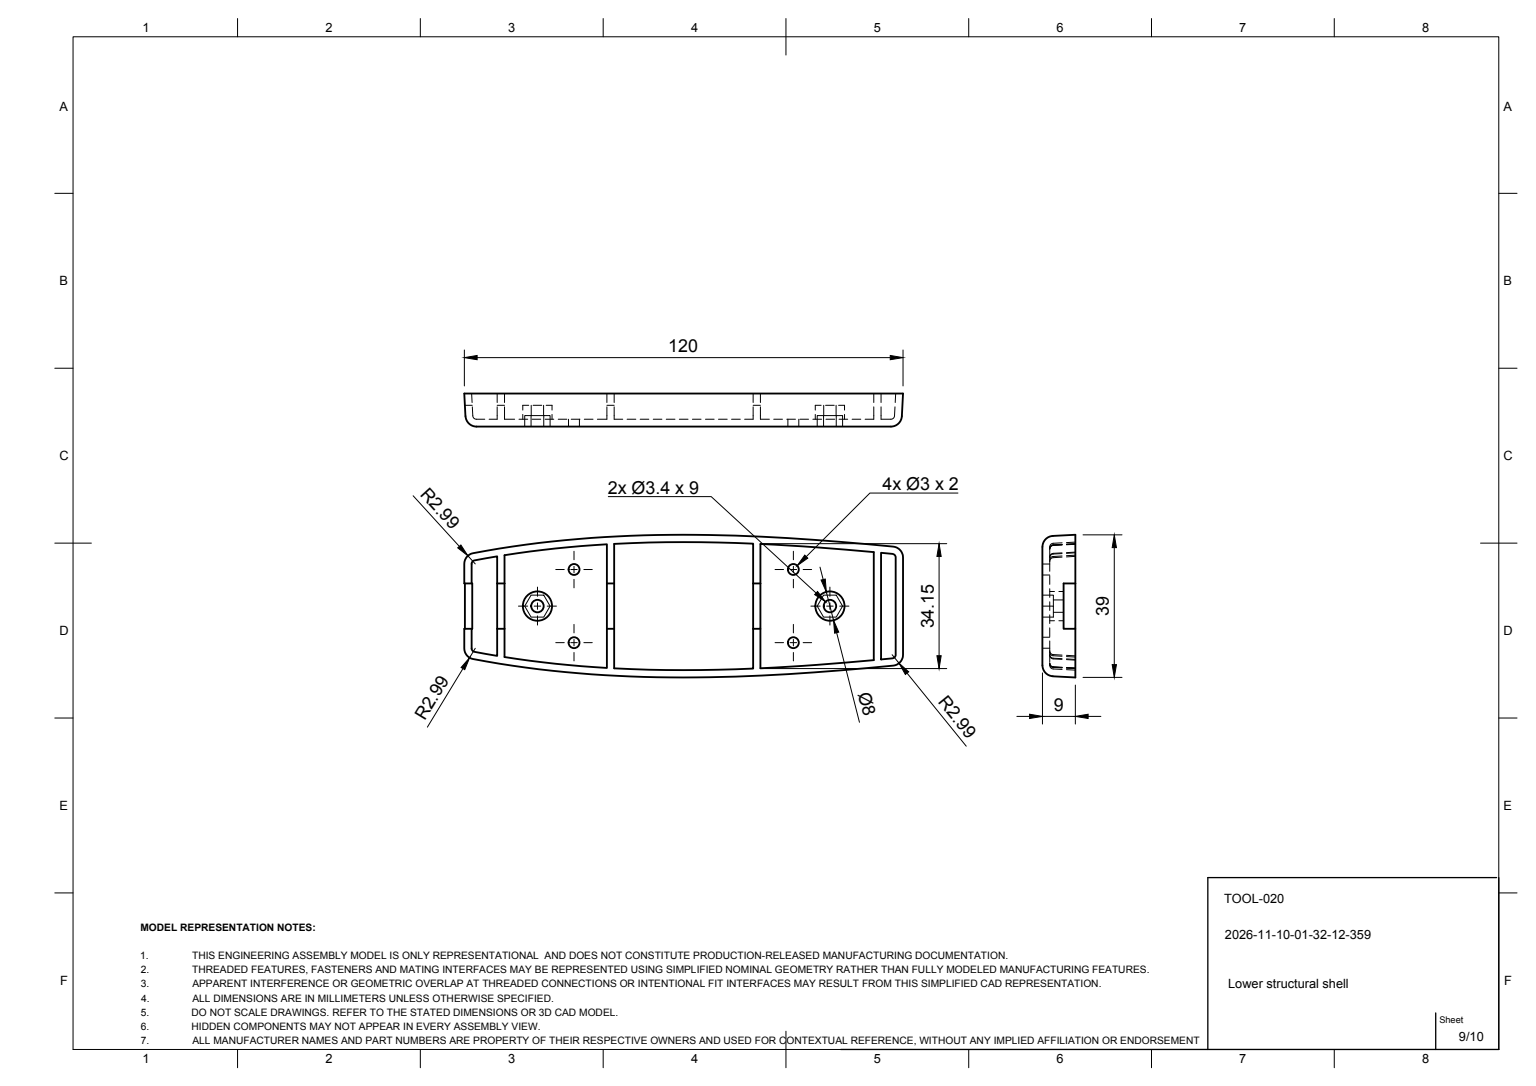
ISO-10303-21;
HEADER;
/* Generated by software containing ST-Developer
 * from STEP Tools, Inc. (www.steptools.com) 
 */

FILE_DESCRIPTION(
/* description */ (''),
/* implementation_level */ '2;1');

FILE_NAME(
/* name */ 'Lower structural shell.step',
/* time_stamp */ '2026-11-10T09:09:39-08:00',
/* author */ (''),
/* organization */ (''),
/* preprocessor_version */ 'ST-DEVELOPER v20.2',
/* originating_system */ 'Autodesk Translation Framework v15.17.0.0',
/* authorisation */ '');

FILE_SCHEMA (('AUTOMOTIVE_DESIGN { 1 0 10303 214 3 1 1 }'));
ENDSEC;

DATA;
#10=MECHANICAL_DESIGN_GEOMETRIC_PRESENTATION_REPRESENTATION('',(#559),#18353);
#83=SPHERICAL_SURFACE('',#6859,0.0999999999999999);
#84=SPHERICAL_SURFACE('',#6862,0.100000000000002);
#85=SPHERICAL_SURFACE('',#6866,0.0999999999999991);
#86=SPHERICAL_SURFACE('',#6870,0.1);
#87=SPHERICAL_SURFACE('',#6875,0.3);
#88=SPHERICAL_SURFACE('',#6879,0.300000000000002);
#89=SPHERICAL_SURFACE('',#6883,0.299999999999999);
#90=SPHERICAL_SURFACE('',#6888,0.3);
#123=B_SPLINE_SURFACE_WITH_KNOTS('',3,3,((#11565,#11566,#11567,#11568),
(#11569,#11570,#11571,#11572),(#11573,#11574,#11575,#11576),(#11577,#11578,
#11579,#11580)),.UNSPECIFIED.,.F.,.F.,.F.,(4,4),(4,4),(0.0627625298587661,
0.3242096015809),(0.0118073085896899,0.685451490706028),.UNSPECIFIED.);
#124=B_SPLINE_SURFACE_WITH_KNOTS('',3,3,((#11585,#11586,#11587,#11588),
(#11589,#11590,#11591,#11592),(#11593,#11594,#11595,#11596),(#11597,#11598,
#11599,#11600)),.UNSPECIFIED.,.F.,.F.,.F.,(4,4),(4,4),(0.0225360950145449,
0.0483865590996774),(0.0125659096559557,0.685650832343257),
 .UNSPECIFIED.);
#125=B_SPLINE_SURFACE_WITH_KNOTS('',3,3,((#11610,#11611,#11612,#11613),
(#11614,#11615,#11616,#11617),(#11618,#11619,#11620,#11621),(#11622,#11623,
#11624,#11625),(#11626,#11627,#11628,#11629)),.UNSPECIFIED.,.F.,.F.,.F.,
(4,1,4),(4,4),(0.,0.571428571428571,1.),(0.74118252158834,3.85438678954986),
 .UNSPECIFIED.);
#126=B_SPLINE_SURFACE_WITH_KNOTS('',3,3,((#11634,#11635,#11636,#11637),
(#11638,#11639,#11640,#11641),(#11642,#11643,#11644,#11645),(#11646,#11647,
#11648,#11649),(#11650,#11651,#11652,#11653)),.UNSPECIFIED.,.F.,.F.,.F.,
(4,1,4),(4,4),(0.,0.571428571428571,1.),(0.270878787657975,0.54981857912664),
 .UNSPECIFIED.);
#127=B_SPLINE_SURFACE_WITH_KNOTS('',3,3,((#11672,#11673,#11674,#11675),
(#11676,#11677,#11678,#11679),(#11680,#11681,#11682,#11683),(#11684,#11685,
#11686,#11687),(#11688,#11689,#11690,#11691)),.UNSPECIFIED.,.F.,.F.,.F.,
(4,1,4),(4,4),(0.,0.571428571428571,1.),(8.03948512627517,11.1526893942367),
 .UNSPECIFIED.);
#128=B_SPLINE_SURFACE_WITH_KNOTS('',3,3,((#11696,#11697,#11698,#11699),
(#11700,#11701,#11702,#11703),(#11704,#11705,#11706,#11707),(#11708,#11709,
#11710,#11711)),.UNSPECIFIED.,.F.,.F.,.F.,(4,4),(4,4),(0.675790398419059,
0.937237470141233),(0.0118073085603101,0.685451490706029),.UNSPECIFIED.);
#129=B_SPLINE_SURFACE_WITH_KNOTS('',3,3,((#11712,#11713,#11714,#11715),
(#11716,#11717,#11718,#11719),(#11720,#11721,#11722,#11723),(#11724,#11725,
#11726,#11727)),.UNSPECIFIED.,.F.,.F.,.F.,(4,4),(4,4),(0.951613440900322,
0.977463904985455),(0.0125659096559558,0.685650832343257),.UNSPECIFIED.);
#130=B_SPLINE_SURFACE_WITH_KNOTS('',3,3,((#11811,#11812,#11813,#11814),
(#11815,#11816,#11817,#11818),(#11819,#11820,#11821,#11822),(#11823,#11824,
#11825,#11826)),.UNSPECIFIED.,.F.,.F.,.F.,(4,4),(4,4),(0.340089900275858,
0.660082688299826),(0.0116294244283504,0.684384408933581),.UNSPECIFIED.);
#131=B_SPLINE_SURFACE_WITH_KNOTS('',3,3,((#11831,#11832,#11833,#11834),
(#11835,#11836,#11837,#11838),(#11839,#11840,#11841,#11842),(#11843,#11844,
#11845,#11846),(#11847,#11848,#11849,#11850)),.UNSPECIFIED.,.F.,.F.,.F.,
(4,1,4),(4,4),(0.,0.571428571428571,1.),(4.04989375377528,7.85140214144331),
 .UNSPECIFIED.);
#132=B_SPLINE_SURFACE_WITH_KNOTS('',3,3,((#11860,#11861,#11862,#11863),
(#11864,#11865,#11866,#11867),(#11868,#11869,#11870,#11871),(#11872,#11873,
#11874,#11875),(#11876,#11877,#11878,#11879)),.UNSPECIFIED.,.F.,.F.,.F.,
(4,1,4),(4,4),(0.,0.571428571428571,1.),(4.0424697743818,7.84397816204974),
 .UNSPECIFIED.);
#133=B_SPLINE_SURFACE_WITH_KNOTS('',3,3,((#11884,#11885,#11886,#11887),
(#11888,#11889,#11890,#11891),(#11892,#11893,#11894,#11895),(#11896,#11897,
#11898,#11899)),.UNSPECIFIED.,.F.,.F.,.F.,(4,4),(4,4),(0.339917311700174,
0.659910099724142),(0.0116294573698948,0.684384408933581),.UNSPECIFIED.);
#134=B_SPLINE_SURFACE_WITH_KNOTS('',3,3,((#11974,#11975,#11976,#11977),
(#11978,#11979,#11980,#11981),(#11982,#11983,#11984,#11985),(#11986,#11987,
#11988,#11989)),.UNSPECIFIED.,.F.,.F.,.F.,(4,4),(4,4),(0.675996615945502,
0.913173856075534),(0.0118505108223707,0.686152089762332),.UNSPECIFIED.);
#135=B_SPLINE_SURFACE_WITH_KNOTS('',3,3,((#11994,#11995,#11996,#11997),
(#11998,#11999,#12000,#12001),(#12002,#12003,#12004,#12005),(#12006,#12007,
#12008,#12009),(#12010,#12011,#12012,#12013)),.UNSPECIFIED.,.F.,.F.,.F.,
(4,1,4),(4,4),(0.,0.571428571428571,1.),(8.0457708503995,10.8690635835914),
 .UNSPECIFIED.);
#136=B_SPLINE_SURFACE_WITH_KNOTS('',3,3,((#12023,#12024,#12025,#12026),
(#12027,#12028,#12029,#12030),(#12031,#12032,#12033,#12034),(#12035,#12036,
#12037,#12038),(#12039,#12040,#12041,#12042)),.UNSPECIFIED.,.F.,.F.,.F.,
(4,1,4),(4,4),(0.,0.571428571428571,1.),(1.02480833223363,3.8481010654256),
 .UNSPECIFIED.);
#137=B_SPLINE_SURFACE_WITH_KNOTS('',3,3,((#12047,#12048,#12049,#12050),
(#12051,#12052,#12053,#12054),(#12055,#12056,#12057,#12058),(#12059,#12060,
#12061,#12062)),.UNSPECIFIED.,.F.,.F.,.F.,(4,4),(4,4),(0.0868261439244655,
0.324003384054498),(0.0118505108223707,0.686152089762332),.UNSPECIFIED.);
#138=B_SPLINE_SURFACE_WITH_KNOTS('',3,3,((#12137,#12138,#12139,#12140),
(#12141,#12142,#12143,#12144),(#12145,#12146,#12147,#12148),(#12149,#12150,
#12151,#12152)),.UNSPECIFIED.,.F.,.F.,.F.,(4,4),(4,4),(0.927751606342899,
0.979699913047832),(0.0130895688562318,0.686930956013783),.UNSPECIFIED.);
#139=B_SPLINE_SURFACE_WITH_KNOTS('',3,3,((#12162,#12163,#12164,#12165),
(#12166,#12167,#12168,#12169),(#12170,#12171,#12172,#12173),(#12174,#12175,
#12176,#12177),(#12178,#12179,#12180,#12181)),.UNSPECIFIED.,.F.,.F.,.F.,
(4,1,4),(4,4),(0.,0.571428571428571,1.),(11.0550486447215,11.6488871259622),
 .UNSPECIFIED.);
#140=B_SPLINE_SURFACE_WITH_KNOTS('',3,3,((#12195,#12196,#12197,#12198),
(#12199,#12200,#12201,#12202),(#12203,#12204,#12205,#12206),(#12207,#12208,
#12209,#12210)),.UNSPECIFIED.,.F.,.F.,.F.,(4,4),(4,4),(0.0203000869521683,
0.0722483936571013),(0.0130895688562318,0.686930956013783),
 .UNSPECIFIED.);
#141=B_SPLINE_SURFACE_WITH_KNOTS('',3,3,((#12220,#12221,#12222,#12223),
(#12224,#12225,#12226,#12227),(#12228,#12229,#12230,#12231),(#12232,#12233,
#12234,#12235),(#12236,#12237,#12238,#12239)),.UNSPECIFIED.,.F.,.F.,.F.,
(4,1,4),(4,4),(0.,0.571428571428571,1.),(0.244984789862841,0.838823271103535),
 .UNSPECIFIED.);
#142=B_SPLINE_SURFACE_WITH_KNOTS('',3,3,((#12253,#12254,#12255,#12256),
(#12257,#12258,#12259,#12260),(#12261,#12262,#12263,#12264),(#12265,#12266,
#12267,#12268),(#12269,#12270,#12271,#12272)),.UNSPECIFIED.,.F.,.F.,.F.,
(4,1,4),(4,4),(0.,0.5,1.),(0.0108921325678979,0.619909717328002),
 .UNSPECIFIED.);
#143=B_SPLINE_SURFACE_WITH_KNOTS('',3,3,((#12279,#12280,#12281,#12282),
(#12283,#12284,#12285,#12286),(#12287,#12288,#12289,#12290),(#12291,#12292,
#12293,#12294),(#12295,#12296,#12297,#12298)),.UNSPECIFIED.,.F.,.F.,.F.,
(4,1,4),(4,4),(0.,0.571428571428571,1.),(0.00967450486392679,0.618764321025346),
 .UNSPECIFIED.);
#144=B_SPLINE_SURFACE_WITH_KNOTS('',3,3,((#12303,#12304,#12305,#12306),
(#12307,#12308,#12309,#12310),(#12311,#12312,#12313,#12314),(#12315,#12316,
#12317,#12318),(#12319,#12320,#12321,#12322)),.UNSPECIFIED.,.F.,.F.,.F.,
(4,1,4),(4,4),(0.,0.571428571428571,1.),(0.0097274579809394,0.618764321025346),
 .UNSPECIFIED.);
#145=B_SPLINE_SURFACE_WITH_KNOTS('',3,3,((#12327,#12328,#12329,#12330),
(#12331,#12332,#12333,#12334),(#12335,#12336,#12337,#12338),(#12339,#12340,
#12341,#12342),(#12343,#12344,#12345,#12346)),.UNSPECIFIED.,.F.,.F.,.F.,
(4,1,4),(4,4),(0.,0.571428571428571,1.),(11.3440533366984,11.6229931281671),
 .UNSPECIFIED.);
#146=B_SPLINE_SURFACE_WITH_KNOTS('',3,3,((#12347,#12348,#12349,#12350),
(#12351,#12352,#12353,#12354),(#12355,#12356,#12357,#12358),(#12359,#12360,
#12361,#12362),(#12363,#12364,#12365,#12366)),.UNSPECIFIED.,.F.,.F.,.F.,
(4,1,4),(4,4),(0.,0.5,1.),(0.0108402259132964,0.619909717328002),
 .UNSPECIFIED.);
#147=B_SPLINE_SURFACE_WITH_KNOTS('',3,3,((#12392,#12393,#12394,#12395),
(#12396,#12397,#12398,#12399),(#12400,#12401,#12402,#12403),(#12404,#12405,
#12406,#12407),(#12408,#12409,#12410,#12411)),.UNSPECIFIED.,.F.,.F.,.F.,
(4,1,4),(4,4),(0.,0.571428571428571,1.),(-0.00387706229521417,0.619909717328002),
 .UNSPECIFIED.);
#148=B_SPLINE_SURFACE_WITH_KNOTS('',3,3,((#12430,#12431,#12432,#12433,#12434,
#12435),(#12436,#12437,#12438,#12439,#12440,#12441),(#12442,#12443,#12444,
#12445,#12446,#12447),(#12448,#12449,#12450,#12451,#12452,#12453),(#12454,
#12455,#12456,#12457,#12458,#12459)),.UNSPECIFIED.,.F.,.F.,.F.,(4,1,4),
(4,1,1,4),(0.,0.571428571428571,1.),(0.270878787657975,5.14716807550265,
8.39802760073243,11.6488871259622),.UNSPECIFIED.);
#149=B_SPLINE_SURFACE_WITH_KNOTS('',3,3,((#12472,#12473,#12474,#12475),
(#12476,#12477,#12478,#12479),(#12480,#12481,#12482,#12483),(#12484,#12485,
#12486,#12487),(#12488,#12489,#12490,#12491)),.UNSPECIFIED.,.F.,.F.,.F.,
(4,1,4),(4,4),(0.,0.571428571428571,1.),(-0.00522825793187074,0.618764321025346),
 .UNSPECIFIED.);
#150=B_SPLINE_SURFACE_WITH_KNOTS('',3,3,((#12500,#12501,#12502,#12503),
(#12504,#12505,#12506,#12507),(#12508,#12509,#12510,#12511),(#12512,#12513,
#12514,#12515),(#12516,#12517,#12518,#12519)),.UNSPECIFIED.,.F.,.F.,.F.,
(4,1,4),(4,4),(0.,0.571428571428571,1.),(-0.00506942997988007,0.618764321025346),
 .UNSPECIFIED.);
#151=B_SPLINE_SURFACE_WITH_KNOTS('',3,3,((#12528,#12529,#12530,#12531,#12532),
(#12533,#12534,#12535,#12536,#12537),(#12538,#12539,#12540,#12541,#12542),
(#12543,#12544,#12545,#12546,#12547),(#12548,#12549,#12550,#12551,#12552)),
 .UNSPECIFIED.,.F.,.F.,.F.,(4,1,4),(4,1,4),(0.,0.571428571428571,1.),(0.244984789862841,
5.12127407770751,11.6229931281671),.UNSPECIFIED.);
#152=B_SPLINE_SURFACE_WITH_KNOTS('',3,3,((#12563,#12564,#12565,#12566),
(#12567,#12568,#12569,#12570),(#12571,#12572,#12573,#12574),(#12575,#12576,
#12577,#12578),(#12579,#12580,#12581,#12582)),.UNSPECIFIED.,.F.,.F.,.F.,
(4,1,4),(4,4),(0.,0.571428571428571,1.),(-0.00403278922781227,0.619909717328002),
 .UNSPECIFIED.);
#153=B_SPLINE_SURFACE_WITH_KNOTS('',3,3,((#12591,#12592,#12593,#12594),
(#12595,#12596,#12597,#12598),(#12599,#12600,#12601,#12602),(#12603,#12604,
#12605,#12606)),.UNSPECIFIED.,.F.,.F.,.F.,(4,4),(4,4),(0.0225340877622934,
0.979701609653785),(0.,0.686930956013783),.UNSPECIFIED.);
#154=B_SPLINE_SURFACE_WITH_KNOTS('',3,3,((#12609,#12610,#12611,#12612),
(#12613,#12614,#12615,#12616),(#12617,#12618,#12619,#12620),(#12621,#12622,
#12623,#12624)),.UNSPECIFIED.,.F.,.F.,.F.,(4,4),(4,4),(0.0202983903462145,
0.977465912237707),(0.,0.686930956013783),.UNSPECIFIED.);
#263=B_SPLINE_CURVE_WITH_KNOTS('',3,(#10837,#10838,#10839,#10840,#10841,
#10842),.UNSPECIFIED.,.F.,.F.,(4,2,4),(-0.607240122656937,-0.303691721894415,
-0.000634514333697656),.UNSPECIFIED.);
#264=B_SPLINE_CURVE_WITH_KNOTS('',3,(#10844,#10845,#10846,#10847,#10848,
#10849,#10850,#10851,#10852,#10853,#10854,#10855,#10856,#10857,#10858,#10859,
#10860,#10861,#10862,#10863,#10864,#10865,#10866,#10867,#10868,#10869,#10870,
#10871),.UNSPECIFIED.,.F.,.F.,(4,3,3,3,3,3,3,3,3,4),(-0.152223584381152,
-0.128403685910756,-0.115058138924018,-0.0911105876986024,-0.0779275105489685,
-0.0651650823668383,-0.0413494676927402,-0.0389105926748606,-0.0151313403168948,
0.),.UNSPECIFIED.);
#265=B_SPLINE_CURVE_WITH_KNOTS('',3,(#10875,#10876,#10877,#10878,#10879,
#10880,#10881,#10882,#10883,#10884,#10885,#10886,#10887,#10888,#10889,#10890,
#10891,#10892,#10893,#10894,#10895,#10896,#10897,#10898,#10899,#10900,#10901,
#10902),.UNSPECIFIED.,.F.,.F.,(4,3,3,3,3,3,3,3,3,4),(-0.152249917238265,
-0.128484865669312,-0.115494642307313,-0.0916985948709881,-0.0870953287403626,
-0.0787006597758974,-0.0547717013112817,-0.0393956522318865,-0.0155460991587222,
0.),.UNSPECIFIED.);
#266=B_SPLINE_CURVE_WITH_KNOTS('',3,(#10903,#10904,#10905,#10906,#10907,
#10908),.UNSPECIFIED.,.F.,.F.,(4,2,4),(-0.606785315485727,-0.30369188913634,
-0.000179692314978108),.UNSPECIFIED.);
#267=B_SPLINE_CURVE_WITH_KNOTS('',3,(#10913,#10914,#10915,#10916,#10917,
#10918),.UNSPECIFIED.,.F.,.F.,(4,2,4),(-0.606332812995025,-0.303737653350621,
-0.000161665236032726),.UNSPECIFIED.);
#268=B_SPLINE_CURVE_WITH_KNOTS('',3,(#10920,#10921,#10922,#10923,#10924,
#10925,#10926,#10927,#10928,#10929,#10930,#10931,#10932,#10933,#10934,#10935,
#10936,#10937,#10938,#10939,#10940,#10941,#10942,#10943,#10944,#10945,#10946,
#10947),.UNSPECIFIED.,.F.,.F.,(4,3,3,3,3,3,3,3,3,4),(-0.152301160038588,
-0.128555435257278,-0.115184785848022,-0.0912639339035621,-0.0780773216554274,
-0.065267350293706,-0.0414723266145325,-0.0390252168402571,-0.0152374671294611,
0.),.UNSPECIFIED.);
#269=B_SPLINE_CURVE_WITH_KNOTS('',3,(#10951,#10952,#10953,#10954,#10955,
#10956,#10957,#10958,#10959,#10960,#10961,#10962,#10963,#10964,#10965,#10966,
#10967,#10968,#10969,#10970,#10971,#10972,#10973,#10974,#10975,#10976,#10977,
#10978),.UNSPECIFIED.,.F.,.F.,(4,3,3,3,3,3,3,3,3,4),(-0.152307894271445,
-0.128535938708366,-0.115295945509717,-0.0915234088298753,-0.0870575315710991,
-0.0782740392368046,-0.0543664511067997,-0.0391484926712317,-0.0153774171089249,
0.),.UNSPECIFIED.);
#270=B_SPLINE_CURVE_WITH_KNOTS('',3,(#10980,#10981,#10982,#10983,#10984,
#10985),.UNSPECIFIED.,.F.,.F.,(4,2,4),(-0.607315067615316,-0.303737782617996,
-0.00114390098251854),.UNSPECIFIED.);
#271=B_SPLINE_CURVE_WITH_KNOTS('',3,(#10991,#10992,#10993,#10994,#10995,
#10996),.UNSPECIFIED.,.F.,.F.,(4,2,4),(-0.606335618682527,-0.303964064424246,
-0.000163142902895597),.UNSPECIFIED.);
#272=B_SPLINE_CURVE_WITH_KNOTS('',3,(#10998,#10999,#11000,#11001,#11002,
#11003,#11004,#11005,#11006,#11007,#11008,#11009,#11010,#11011,#11012,#11013,
#11014,#11015,#11016,#11017,#11018,#11019,#11020,#11021,#11022,#11023,#11024,
#11025),.UNSPECIFIED.,.F.,.F.,(4,3,3,3,3,3,3,3,3,4),(-0.152324888062519,
-0.128571266282871,-0.115187819092559,-0.0912644922975459,-0.0780623053857969,
-0.0652705430018984,-0.0414736125245103,-0.0390138150290758,-0.015226502089553,
0.),.UNSPECIFIED.);
#273=B_SPLINE_CURVE_WITH_KNOTS('',3,(#11029,#11030,#11031,#11032,#11033,
#11034,#11035,#11036,#11037,#11038,#11039,#11040,#11041,#11042,#11043,#11044,
#11045,#11046,#11047,#11048,#11049,#11050,#11051,#11052,#11053,#11054,#11055,
#11056),.UNSPECIFIED.,.F.,.F.,(4,3,3,3,3,3,3,3,3,4),(-0.152333600285603,
-0.128561769460285,-0.115331525958272,-0.0915566852459163,-0.0870792380259527,
-0.0783165909319309,-0.0544069520497563,-0.0391732033593778,-0.0153939862842036,
0.),.UNSPECIFIED.);
#274=B_SPLINE_CURVE_WITH_KNOTS('',3,(#11058,#11059,#11060,#11061,#11062,
#11063),.UNSPECIFIED.,.F.,.F.,(4,2,4),(-0.607765665607205,-0.303964210965506,
-0.00159316434717749),.UNSPECIFIED.);
#275=B_SPLINE_CURVE_WITH_KNOTS('',3,(#11069,#11070,#11071,#11072,#11073,
#11074),.UNSPECIFIED.,.F.,.F.,(4,2,4),(-0.608113833554089,-0.304405910662044,
-0.00120843896277512),.UNSPECIFIED.);
#276=B_SPLINE_CURVE_WITH_KNOTS('',3,(#11076,#11077,#11078,#11079,#11080,
#11081,#11082,#11083,#11084,#11085,#11086,#11087,#11088,#11089,#11090,#11091,
#11092,#11093,#11094,#11095,#11096,#11097,#11098,#11099,#11100,#11101,#11102,
#11103),.UNSPECIFIED.,.F.,.F.,(4,3,3,3,3,3,3,3,3,4),(-0.152638346832965,
-0.128647829044501,-0.117000727359648,-0.0929750760194364,-0.0775532335837778,
-0.065166230851578,-0.0413072760700971,-0.0386249916896363,-0.0148681833632798,
0.),.UNSPECIFIED.);
#277=B_SPLINE_CURVE_WITH_KNOTS('',3,(#11107,#11108,#11109,#11110,#11111,
#11112,#11113,#11114,#11115,#11116,#11117,#11118,#11119,#11120,#11121,#11122,
#11123,#11124,#11125,#11126,#11127,#11128,#11129,#11130,#11131,#11132,#11133,
#11134),.UNSPECIFIED.,.F.,.F.,(4,3,3,3,3,3,3,3,3,4),(-0.152712908768378,
-0.128963682254188,-0.116304008925778,-0.092453135123643,-0.0875380734791113,
-0.0797852913889514,-0.0558105568475602,-0.0400274901149945,-0.0159798645019078,
0.),.UNSPECIFIED.);
#278=B_SPLINE_CURVE_WITH_KNOTS('',3,(#11136,#11137,#11138,#11139,#11140,
#11141),.UNSPECIFIED.,.F.,.F.,(4,2,4),(-0.607607610897069,-0.304406883675693,
-0.000702187548907163),.UNSPECIFIED.);
#279=B_SPLINE_CURVE_WITH_KNOTS('',3,(#11147,#11148,#11149,#11150),
 .UNSPECIFIED.,.F.,.F.,(4,4),(0.0130288733793136,0.619909717328002),
 .UNSPECIFIED.);
#280=B_SPLINE_CURVE_WITH_KNOTS('',3,(#11154,#11155,#11156,#11157),
 .UNSPECIFIED.,.F.,.F.,(4,4),(-0.619909717328002,-0.0130288733793137),
 .UNSPECIFIED.);
#281=B_SPLINE_CURVE_WITH_KNOTS('',3,(#11160,#11161,#11162,#11163,#11164,
#11165,#11166),.UNSPECIFIED.,.F.,.F.,(4,3,4),(7.87274532319472,10.4298004347969,
10.9780233963721),.UNSPECIFIED.);
#282=B_SPLINE_CURVE_WITH_KNOTS('',3,(#11167,#11168,#11169,#11170,#11171,
#11172,#11173),.UNSPECIFIED.,.F.,.F.,(4,3,4),(0.511752108249611,2.84807862798167,
3.61537599721027),.UNSPECIFIED.);
#283=B_SPLINE_CURVE_WITH_KNOTS('',3,(#11176,#11177,#11178,#11179,#11180,
#11181,#11182),.UNSPECIFIED.,.F.,.F.,(4,3,4),(3.81523717927831,5.72635044542746,
7.61820606472736),.UNSPECIFIED.);
#284=B_SPLINE_CURVE_WITH_KNOTS('',3,(#11185,#11186,#11187,#11188),
 .UNSPECIFIED.,.F.,.F.,(4,4),(7.8195516254834,10.6519234170402),
 .UNSPECIFIED.);
#285=B_SPLINE_CURVE_WITH_KNOTS('',3,(#11192,#11193,#11194,#11195),
 .UNSPECIFIED.,.F.,.F.,(4,4),(10.8550709503701,11.4839159448819),
 .UNSPECIFIED.);
#286=B_SPLINE_CURVE_WITH_KNOTS('',3,(#11196,#11197,#11198,#11199,#11200,
#11201,#11202,#11203,#11204,#11205,#11206,#11207,#11208,#11209,#11210,#11211,
#11212,#11213,#11214,#11215,#11216,#11217,#11218,#11219,#11220,#11221,#11222,
#11223),.UNSPECIFIED.,.F.,.F.,(4,3,3,3,3,3,3,3,3,4),(0.,0.023800266251022,
0.0390470051780055,0.062864594207143,0.0692752090304052,0.0780196763370091,
0.101808338076191,0.108235461704482,0.131970324379069,0.138468980573541),
 .UNSPECIFIED.);
#287=B_SPLINE_CURVE_WITH_KNOTS('',3,(#11227,#11228,#11229,#11230,#11231,
#11232,#11233,#11234,#11235,#11236,#11237,#11238,#11239,#11240,#11241,#11242,
#11243,#11244,#11245,#11246,#11247,#11248,#11249,#11250,#11251,#11252,#11253,
#11254,#11255,#11256,#11257),.UNSPECIFIED.,.F.,.F.,(4,3,3,3,3,3,3,3,3,3,
4),(0.,0.0536158767337707,0.107707970980176,0.117140678528723,0.171373940961503,
0.178118425384842,0.234058785038521,0.2884659822146,0.324708667187819,0.378759781373182,
0.415412568437851),.UNSPECIFIED.);
#288=B_SPLINE_CURVE_WITH_KNOTS('',3,(#11259,#11260,#11261,#11262),
 .UNSPECIFIED.,.F.,.F.,(4,4),(0.0202983903462145,0.977465912237707),
 .UNSPECIFIED.);
#289=B_SPLINE_CURVE_WITH_KNOTS('',3,(#11264,#11265,#11266,#11267,#11268,
#11269,#11270,#11271,#11272,#11273,#11274,#11275,#11276,#11277,#11278,#11279,
#11280,#11281,#11282,#11283,#11284,#11285,#11286,#11287,#11288,#11289,#11290,
#11291,#11292,#11293,#11294),.UNSPECIFIED.,.F.,.F.,(4,3,3,3,3,3,3,3,3,3,
4),(0.,0.053547205187505,0.107728964525782,0.117299670245694,0.171524652009909,
0.189842726242433,0.234296321023441,0.288773621215207,0.338477936388461,
0.392564001789548,0.442713223041249),.UNSPECIFIED.);
#290=B_SPLINE_CURVE_WITH_KNOTS('',3,(#11298,#11299,#11300,#11301,#11302,
#11303,#11304,#11305,#11306,#11307,#11308,#11309,#11310,#11311,#11312,#11313,
#11314,#11315,#11316,#11317,#11318,#11319,#11320,#11321,#11322,#11323,#11324,
#11325,#11326,#11327,#11328),.UNSPECIFIED.,.F.,.F.,(4,3,3,3,3,3,3,3,3,3,
4),(0.,0.0535312152416108,0.107707123412492,0.117215931328448,0.171445047002381,
0.189808362521926,0.234165405003858,0.288639615809812,0.338404447092272,
0.392504428396833,0.442708851597914),.UNSPECIFIED.);
#291=B_SPLINE_CURVE_WITH_KNOTS('',3,(#11330,#11331,#11332,#11333),
 .UNSPECIFIED.,.F.,.F.,(4,4),(0.0225340877622936,0.979701609653785),
 .UNSPECIFIED.);
#292=B_SPLINE_CURVE_WITH_KNOTS('',3,(#11335,#11336,#11337,#11338,#11339,
#11340,#11341,#11342,#11343,#11344,#11345,#11346,#11347,#11348,#11349,#11350,
#11351,#11352,#11353,#11354,#11355,#11356,#11357,#11358,#11359,#11360,#11361,
#11362,#11363,#11364,#11365),.UNSPECIFIED.,.F.,.F.,(4,3,3,3,3,3,3,3,3,3,
4),(0.,0.0536458552170769,0.107744721567334,0.117297895480617,0.171522683869793,
0.178177673384308,0.23429412186666,0.288702228477357,0.324838815929715,
0.378862861687027,0.415420074045746),.UNSPECIFIED.);
#293=B_SPLINE_CURVE_WITH_KNOTS('',3,(#11368,#11369,#11370,#11371,#11372,
#11373,#11374,#11375,#11376,#11377,#11378,#11379,#11380,#11381,#11382,#11383,
#11384,#11385,#11386,#11387,#11388,#11389,#11390,#11391,#11392,#11393,#11394,
#11395),.UNSPECIFIED.,.F.,.F.,(4,3,3,3,3,3,3,3,3,4),(0.,0.0238098951475563,
0.0390995920428052,0.0629117710415135,0.0692953339558167,0.0780985718814299,
0.101889748471939,0.108278926258091,0.132003149848588,0.138471484390145),
 .UNSPECIFIED.);
#294=B_SPLINE_CURVE_WITH_KNOTS('',3,(#11397,#11398,#11399,#11400),
 .UNSPECIFIED.,.F.,.F.,(4,4),(2.05597917304345E-5,0.629200412657851),
 .UNSPECIFIED.);
#295=B_SPLINE_CURVE_WITH_KNOTS('',3,(#11403,#11404,#11405,#11406),
 .UNSPECIFIED.,.F.,.F.,(4,4),(0.832456091119126,3.6663340257767),
 .UNSPECIFIED.);
#296=B_SPLINE_CURVE_WITH_KNOTS('',3,(#11409,#11410,#11411,#11412,#11413,
#11414,#11415),.UNSPECIFIED.,.F.,.F.,(4,3,4),(3.86778652923942,5.76006783397632,
7.67277763234621),.UNSPECIFIED.);
#297=B_SPLINE_CURVE_WITH_KNOTS('',3,(#11419,#11420,#11421,#11422),
 .UNSPECIFIED.,.F.,.F.,(4,4),(11.1789026308149,11.490024089745),
 .UNSPECIFIED.);
#298=B_SPLINE_CURVE_WITH_KNOTS('',3,(#11424,#11425,#11426,#11427,#11428,
#11429,#11430,#11431,#11432,#11433,#11434,#11435,#11436,#11437,#11438,#11439,
#11440,#11441,#11442,#11443,#11444,#11445,#11446,#11447,#11448),
 .UNSPECIFIED.,.F.,.F.,(4,3,3,3,3,3,3,3,4),(0.,0.0238050540413609,0.0390723036702896,
0.0632692088215501,0.0780555758269344,0.101951849921082,0.112801451778717,
0.136536488207902,0.147568670144067),.UNSPECIFIED.);
#299=B_SPLINE_CURVE_WITH_KNOTS('',3,(#11452,#11453,#11454,#11455,#11456,
#11457,#11458,#11459,#11460,#11461,#11462,#11463,#11464,#11465,#11466,#11467,
#11468,#11469,#11470,#11471,#11472,#11473,#11474,#11475,#11476),
 .UNSPECIFIED.,.F.,.F.,(4,3,3,3,3,3,3,3,4),(0.,0.0238098889950854,0.0391003179068551,
0.0632803937136523,0.0780994777107358,0.101997157448698,0.112825962756833,
0.136555142506291,0.147570127973408),.UNSPECIFIED.);
#300=B_SPLINE_CURVE_WITH_KNOTS('',3,(#11478,#11479,#11480,#11481),
 .UNSPECIFIED.,.F.,.F.,(4,4),(2.41556456535008E-5,0.310979882704647),
 .UNSPECIFIED.);
#301=B_SPLINE_CURVE_WITH_KNOTS('',3,(#11493,#11494,#11495,#11496,#11497,
#11498),.UNSPECIFIED.,.F.,.F.,(4,2,4),(-0.606744425054929,-0.30369469419025,
-0.000104868936493974),.UNSPECIFIED.);
#302=B_SPLINE_CURVE_WITH_KNOTS('',3,(#11500,#11501,#11502,#11503,#11504,
#11505),.UNSPECIFIED.,.F.,.F.,(4,2,4),(-0.60732337425873,-0.303694522808999,
-0.000683832228057069),.UNSPECIFIED.);
#303=B_SPLINE_CURVE_WITH_KNOTS('',3,(#11507,#11508,#11509,#11510,#11511,
#11512,#11513,#11514,#11515,#11516,#11517,#11518,#11519,#11520,#11521,#11522,
#11523,#11524,#11525,#11526,#11527,#11528,#11529,#11530,#11531,#11532,#11533,
#11534),.UNSPECIFIED.,.F.,.F.,(4,3,3,3,3,3,3,3,3,4),(-0.152213081758773,
-0.128388856548194,-0.115047734630008,-0.0910986092737131,-0.0779187269986961,
-0.0651565114518209,-0.0413397067626705,-0.0389038209724845,-0.0151251319644201,
0.),.UNSPECIFIED.);
#304=B_SPLINE_CURVE_WITH_KNOTS('',3,(#11537,#11538,#11539,#11540,#11541,
#11542,#11543,#11544,#11545,#11546,#11547,#11548,#11549,#11550,#11551,#11552,
#11553,#11554,#11555,#11556,#11557,#11558,#11559,#11560,#11561,#11562,#11563,
#11564),.UNSPECIFIED.,.F.,.F.,(4,3,3,3,3,3,3,3,3,4),(-0.152240567100014,
-0.128476012965191,-0.115503482174674,-0.0917060839439778,-0.0870941983819305,
-0.0787260045726768,-0.0547958477503903,-0.0394103419198022,-0.0155561788900784,
0.),.UNSPECIFIED.);
#305=B_SPLINE_CURVE_WITH_KNOTS('',3,(#11581,#11582,#11583,#11584),
 .UNSPECIFIED.,.F.,.F.,(4,4),(-3.85438678954986,-0.750511952447855),
 .UNSPECIFIED.);
#306=B_SPLINE_CURVE_WITH_KNOTS('',3,(#11602,#11603,#11604,#11605),
 .UNSPECIFIED.,.F.,.F.,(4,4),(-0.54981857912664,-0.270878787657975),
 .UNSPECIFIED.);
#307=B_SPLINE_CURVE_WITH_KNOTS('',3,(#11606,#11607,#11608,#11609),
 .UNSPECIFIED.,.F.,.F.,(4,4),(-0.618764321025346,-0.0114172178585034),
 .UNSPECIFIED.);
#308=B_SPLINE_CURVE_WITH_KNOTS('',3,(#11630,#11631,#11632,#11633),
 .UNSPECIFIED.,.F.,.F.,(4,4),(0.74118252158834,3.84969085360113),
 .UNSPECIFIED.);
#309=B_SPLINE_CURVE_WITH_KNOTS('',3,(#11655,#11656,#11657,#11658),
 .UNSPECIFIED.,.F.,.F.,(4,4),(0.270878787657975,0.540284107299618),
 .UNSPECIFIED.);
#310=B_SPLINE_CURVE_WITH_KNOTS('',3,(#11661,#11662,#11663,#11664),
 .UNSPECIFIED.,.F.,.F.,(4,4),(8.04418106222393,11.1526893942367),
 .UNSPECIFIED.);
#311=B_SPLINE_CURVE_WITH_KNOTS('',3,(#11667,#11668,#11669,#11670),
 .UNSPECIFIED.,.F.,.F.,(4,4),(11.3535878085254,11.6229931281671),
 .UNSPECIFIED.);
#312=B_SPLINE_CURVE_WITH_KNOTS('',3,(#11692,#11693,#11694,#11695),
 .UNSPECIFIED.,.F.,.F.,(4,4),(-11.1433599633772,-8.03948512627517),
 .UNSPECIFIED.);
#313=B_SPLINE_CURVE_WITH_KNOTS('',3,(#11729,#11730,#11731,#11732),
 .UNSPECIFIED.,.F.,.F.,(4,4),(0.0114172178585033,0.618764321025346),
 .UNSPECIFIED.);
#314=B_SPLINE_CURVE_WITH_KNOTS('',3,(#11733,#11734,#11735,#11736),
 .UNSPECIFIED.,.F.,.F.,(4,4),(-11.6229931281671,-11.3440533366984),
 .UNSPECIFIED.);
#315=B_SPLINE_CURVE_WITH_KNOTS('',3,(#11739,#11740,#11741,#11742,#11743,
#11744),.UNSPECIFIED.,.F.,.F.,(4,2,4),(-0.606286853269513,-0.303735636734938,
-0.000134370544016882),.UNSPECIFIED.);
#316=B_SPLINE_CURVE_WITH_KNOTS('',3,(#11746,#11747,#11748,#11749,#11750,
#11751,#11752,#11753,#11754,#11755,#11756,#11757,#11758,#11759,#11760,#11761,
#11762,#11763,#11764,#11765,#11766,#11767,#11768,#11769,#11770,#11771,#11772,
#11773),.UNSPECIFIED.,.F.,.F.,(4,3,3,3,3,3,3,3,3,4),(-0.152301724526365,
-0.128559761662057,-0.115189905045126,-0.0912708316251271,-0.0780855696141105,
-0.0652713768517459,-0.0414777101816728,-0.0390314967756457,-0.015242903619151,
0.),.UNSPECIFIED.);
#317=B_SPLINE_CURVE_WITH_KNOTS('',3,(#11777,#11778,#11779,#11780,#11781,
#11782,#11783,#11784,#11785,#11786,#11787,#11788,#11789,#11790,#11791,#11792,
#11793,#11794,#11795,#11796,#11797,#11798,#11799,#11800,#11801,#11802,#11803,
#11804),.UNSPECIFIED.,.F.,.F.,(4,3,3,3,3,3,3,3,3,4),(-0.1523073815286,-0.1285346644938,
-0.115283264026726,-0.0915123087981378,-0.0870533687950649,-0.0782507800682277,
-0.0543447803816484,-0.0391350231834537,-0.0153679399182895,0.),
 .UNSPECIFIED.);
#318=B_SPLINE_CURVE_WITH_KNOTS('',3,(#11805,#11806,#11807,#11808,#11809,
#11810),.UNSPECIFIED.,.F.,.F.,(4,2,4),(-0.607338074051965,-0.303735662161239,
-0.00118557149519966),.UNSPECIFIED.);
#319=B_SPLINE_CURVE_WITH_KNOTS('',3,(#11827,#11828,#11829,#11830),
 .UNSPECIFIED.,.F.,.F.,(4,4),(-7.8460657686783,-4.05419673417835),
 .UNSPECIFIED.);
#320=B_SPLINE_CURVE_WITH_KNOTS('',3,(#11851,#11852,#11853,#11854),
 .UNSPECIFIED.,.F.,.F.,(4,4),(4.04989375377528,7.85140214144331),
 .UNSPECIFIED.);
#321=B_SPLINE_CURVE_WITH_KNOTS('',3,(#11856,#11857,#11858,#11859),
 .UNSPECIFIED.,.F.,.F.,(4,4),(4.0424697743818,7.84397816204974),
 .UNSPECIFIED.);
#322=B_SPLINE_CURVE_WITH_KNOTS('',3,(#11880,#11881,#11882,#11883),
 .UNSPECIFIED.,.F.,.F.,(4,4),(-7.83967518164668,-4.0478061471468),
 .UNSPECIFIED.);
#323=B_SPLINE_CURVE_WITH_KNOTS('',3,(#11902,#11903,#11904,#11905,#11906,
#11907),.UNSPECIFIED.,.F.,.F.,(4,2,4),(-0.606398914035431,-0.303967092551845,
-0.000200694235479137),.UNSPECIFIED.);
#324=B_SPLINE_CURVE_WITH_KNOTS('',3,(#11909,#11910,#11911,#11912,#11913,
#11914,#11915,#11916,#11917,#11918,#11919,#11920,#11921,#11922,#11923,#11924,
#11925,#11926,#11927,#11928,#11929,#11930,#11931,#11932,#11933,#11934,#11935,
#11936),.UNSPECIFIED.,.F.,.F.,(4,3,3,3,3,3,3,3,3,4),(-0.15233244131821,
-0.128569871170003,-0.115181988990177,-0.0912564475476021,-0.0780459432968613,
-0.0652662335163151,-0.0414674738832469,-0.0390013640446512,-0.0152139229936509,
0.),.UNSPECIFIED.);
#325=B_SPLINE_CURVE_WITH_KNOTS('',3,(#11940,#11941,#11942,#11943,#11944,
#11945,#11946,#11947,#11948,#11949,#11950,#11951,#11952,#11953,#11954,#11955,
#11956,#11957,#11958,#11959,#11960,#11961,#11962,#11963,#11964,#11965,#11966,
#11967),.UNSPECIFIED.,.F.,.F.,(4,3,3,3,3,3,3,3,3,4),(-0.152343297533924,
-0.128571042154168,-0.115361098257144,-0.0915841820623439,-0.0870924557961151,
-0.0783628838319633,-0.0544516462338148,-0.0392000432438046,-0.0154115240971992,
0.),.UNSPECIFIED.);
#326=B_SPLINE_CURVE_WITH_KNOTS('',3,(#11968,#11969,#11970,#11971,#11972,
#11973),.UNSPECIFIED.,.F.,.F.,(4,2,4),(-0.607734321217702,-0.303967174049374,
-0.00153607519677973),.UNSPECIFIED.);
#327=B_SPLINE_CURVE_WITH_KNOTS('',3,(#11990,#11991,#11992,#11993),
 .UNSPECIFIED.,.F.,.F.,(4,4),(-10.8531956503852,-8.0457708503995),
 .UNSPECIFIED.);
#328=B_SPLINE_CURVE_WITH_KNOTS('',3,(#12014,#12015,#12016,#12017),
 .UNSPECIFIED.,.F.,.F.,(4,4),(8.05172912332209,10.8690635835914),
 .UNSPECIFIED.);
#329=B_SPLINE_CURVE_WITH_KNOTS('',3,(#12019,#12020,#12021,#12022),
 .UNSPECIFIED.,.F.,.F.,(4,4),(1.02480833223363,3.84214279250303),
 .UNSPECIFIED.);
#330=B_SPLINE_CURVE_WITH_KNOTS('',3,(#12043,#12044,#12045,#12046),
 .UNSPECIFIED.,.F.,.F.,(4,4),(-3.8481010654256,-1.04067626543981),
 .UNSPECIFIED.);
#331=B_SPLINE_CURVE_WITH_KNOTS('',3,(#12065,#12066,#12067,#12068,#12069,
#12070),.UNSPECIFIED.,.F.,.F.,(4,2,4),(-0.608301643694891,-0.304416323412316,
-0.0013178649037765),.UNSPECIFIED.);
#332=B_SPLINE_CURVE_WITH_KNOTS('',3,(#12072,#12073,#12074,#12075,#12076,
#12077,#12078,#12079,#12080,#12081,#12082,#12083,#12084,#12085,#12086,#12087,
#12088,#12089,#12090,#12091,#12092,#12093,#12094,#12095,#12096,#12097,#12098,
#12099),.UNSPECIFIED.,.F.,.F.,(4,3,3,3,3,3,3,3,3,4),(-0.152679905805259,
-0.128657903528546,-0.116982385578132,-0.0929502017086943,-0.0774957796939621,
-0.0651567901405441,-0.0412920018136918,-0.0385809476656748,-0.0148252868187304,
0.),.UNSPECIFIED.);
#333=B_SPLINE_CURVE_WITH_KNOTS('',3,(#12103,#12104,#12105,#12106,#12107,
#12108,#12109,#12110,#12111,#12112,#12113,#12114,#12115,#12116,#12117,#12118,
#12119,#12120,#12121,#12122,#12123,#12124,#12125,#12126,#12127,#12128,#12129,
#12130),.UNSPECIFIED.,.F.,.F.,(4,3,3,3,3,3,3,3,3,4),(-0.152762160496458,
-0.129013039804674,-0.116418683706179,-0.0925605502531877,-0.0875939536119484,
-0.0799546107253736,-0.055976748465099,-0.0401263304884301,-0.0160466564276224,
0.),.UNSPECIFIED.);
#334=B_SPLINE_CURVE_WITH_KNOTS('',3,(#12131,#12132,#12133,#12134,#12135,
#12136),.UNSPECIFIED.,.F.,.F.,(4,2,4),(-0.607519387555057,-0.304417308507995,
-0.000535579674449116),.UNSPECIFIED.);
#335=B_SPLINE_CURVE_WITH_KNOTS('',3,(#12154,#12155,#12156,#12157),
 .UNSPECIFIED.,.F.,.F.,(4,4),(0.012184405392802,0.619909717328002),
 .UNSPECIFIED.);
#336=B_SPLINE_CURVE_WITH_KNOTS('',3,(#12158,#12159,#12160,#12161),
 .UNSPECIFIED.,.F.,.F.,(4,4),(-11.6488871259622,-11.0550486447215),
 .UNSPECIFIED.);
#337=B_SPLINE_CURVE_WITH_KNOTS('',3,(#12184,#12185,#12186,#12187),
 .UNSPECIFIED.,.F.,.F.,(4,4),(11.0717103908866,11.6488871259622),
 .UNSPECIFIED.);
#338=B_SPLINE_CURVE_WITH_KNOTS('',3,(#12191,#12192,#12193,#12194),
 .UNSPECIFIED.,.F.,.F.,(4,4),(0.244984789862841,0.822161524938444),
 .UNSPECIFIED.);
#339=B_SPLINE_CURVE_WITH_KNOTS('',3,(#12212,#12213,#12214,#12215),
 .UNSPECIFIED.,.F.,.F.,(4,4),(-0.838823271103535,-0.244984789862841),
 .UNSPECIFIED.);
#340=B_SPLINE_CURVE_WITH_KNOTS('',3,(#12216,#12217,#12218,#12219),
 .UNSPECIFIED.,.F.,.F.,(4,4),(-0.619909717328002,-0.0121844053928019),
 .UNSPECIFIED.);
#341=B_SPLINE_CURVE_WITH_KNOTS('',3,(#12299,#12300,#12301,#12302),
 .UNSPECIFIED.,.F.,.F.,(4,4),(0.011877999214525,0.618764321025346),
 .UNSPECIFIED.);
#342=B_SPLINE_CURVE_WITH_KNOTS('',3,(#12323,#12324,#12325,#12326),
 .UNSPECIFIED.,.F.,.F.,(4,4),(-0.618764321025346,-0.0118779992145249),
 .UNSPECIFIED.);
#343=B_SPLINE_CURVE_WITH_KNOTS('',3,(#12412,#12413,#12414,#12415),
 .UNSPECIFIED.,.F.,.F.,(4,4),(-1.34441069388203E-17,0.619909717328002),
 .UNSPECIFIED.);
#344=B_SPLINE_CURVE_WITH_KNOTS('',3,(#12416,#12417,#12418,#12419),
 .UNSPECIFIED.,.F.,.F.,(4,4),(-0.619909717328002,-0.00253319281730041),
 .UNSPECIFIED.);
#345=B_SPLINE_CURVE_WITH_KNOTS('',3,(#12460,#12461,#12462,#12463,#12464,
#12465),.UNSPECIFIED.,.F.,.F.,(4,1,1,4),(-11.6488871259622,-8.39802760073243,
-5.14716807550265,-0.270878787657975),.UNSPECIFIED.);
#346=B_SPLINE_CURVE_WITH_KNOTS('',3,(#12466,#12467,#12468,#12469,#12470,
#12471),.UNSPECIFIED.,.F.,.F.,(4,1,1,4),(0.270878787657975,5.14716807550265,
8.39802760073243,11.6488871259622),.UNSPECIFIED.);
#347=B_SPLINE_CURVE_WITH_KNOTS('',3,(#12492,#12493,#12494,#12495),
 .UNSPECIFIED.,.F.,.F.,(4,4),(0.0013822243147816,0.618764321025346),
 .UNSPECIFIED.);
#348=B_SPLINE_CURVE_WITH_KNOTS('',3,(#12496,#12497,#12498,#12499),
 .UNSPECIFIED.,.F.,.F.,(4,4),(-0.618764321025346,8.06646416329215E-17),
 .UNSPECIFIED.);
#349=B_SPLINE_CURVE_WITH_KNOTS('',3,(#12520,#12521,#12522,#12523),
 .UNSPECIFIED.,.F.,.F.,(4,4),(-9.36750677027476E-17,0.618764321025346),
 .UNSPECIFIED.);
#350=B_SPLINE_CURVE_WITH_KNOTS('',3,(#12524,#12525,#12526,#12527),
 .UNSPECIFIED.,.F.,.F.,(4,4),(-0.618764321025346,-0.00138222431478148),
 .UNSPECIFIED.);
#351=B_SPLINE_CURVE_WITH_KNOTS('',3,(#12553,#12554,#12555,#12556,#12557),
 .UNSPECIFIED.,.F.,.F.,(4,1,4),(-11.6229931281671,-5.12127407770751,-0.244984789862841),
 .UNSPECIFIED.);
#352=B_SPLINE_CURVE_WITH_KNOTS('',3,(#12558,#12559,#12560,#12561,#12562),
 .UNSPECIFIED.,.F.,.F.,(4,1,4),(0.244984789862841,5.12127407770751,11.6229931281671),
 .UNSPECIFIED.);
#353=B_SPLINE_CURVE_WITH_KNOTS('',3,(#12583,#12584,#12585,#12586),
 .UNSPECIFIED.,.F.,.F.,(4,4),(0.00253319281730024,0.619909717328002),
 .UNSPECIFIED.);
#354=B_SPLINE_CURVE_WITH_KNOTS('',3,(#12587,#12588,#12589,#12590),
 .UNSPECIFIED.,.F.,.F.,(4,4),(-0.619909717328002,-2.51534904016637E-17),
 .UNSPECIFIED.);
#541=SHAPE_REPRESENTATION_RELATIONSHIP('SRR','None',#18402,#550);
#550=ADVANCED_BREP_SHAPE_REPRESENTATION('',(#568),#18348);
#559=STYLED_ITEM('',(#18459),#568);
#568=MANIFOLD_SOLID_BREP('Body1',#6490);
#603=FACE_BOUND('',#1330,.T.);
#604=FACE_BOUND('',#1338,.T.);
#605=FACE_BOUND('',#1349,.T.);
#606=FACE_BOUND('',#1351,.T.);
#607=FACE_BOUND('',#1363,.T.);
#608=FACE_BOUND('',#1372,.T.);
#609=FACE_BOUND('',#1373,.T.);
#610=FACE_BOUND('',#1374,.T.);
#611=FACE_BOUND('',#1389,.T.);
#612=FACE_BOUND('',#1390,.T.);
#613=FACE_BOUND('',#1391,.T.);
#614=FACE_BOUND('',#1427,.T.);
#615=FACE_BOUND('',#1428,.T.);
#616=FACE_BOUND('',#1429,.T.);
#617=FACE_BOUND('',#1430,.T.);
#618=FACE_BOUND('',#1431,.T.);
#619=FACE_BOUND('',#1432,.T.);
#703=PLANE('',#6801);
#704=PLANE('',#6802);
#705=PLANE('',#6803);
#706=PLANE('',#6804);
#707=PLANE('',#6805);
#708=PLANE('',#6806);
#709=PLANE('',#6807);
#710=PLANE('',#6809);
#711=PLANE('',#6810);
#712=PLANE('',#6811);
#713=PLANE('',#6812);
#714=PLANE('',#6813);
#715=PLANE('',#6814);
#716=PLANE('',#6815);
#717=PLANE('',#6821);
#718=PLANE('',#6822);
#719=PLANE('',#6823);
#720=PLANE('',#6824);
#721=PLANE('',#6825);
#722=PLANE('',#6826);
#723=PLANE('',#6827);
#724=PLANE('',#6828);
#725=PLANE('',#6830);
#726=PLANE('',#6832);
#727=PLANE('',#6833);
#728=PLANE('',#6834);
#729=PLANE('',#6835);
#730=PLANE('',#6836);
#731=PLANE('',#6837);
#732=PLANE('',#6838);
#733=PLANE('',#6839);
#734=PLANE('',#6840);
#735=PLANE('',#6841);
#736=PLANE('',#6842);
#737=PLANE('',#6847);
#738=PLANE('',#6849);
#739=PLANE('',#6850);
#740=PLANE('',#6851);
#741=PLANE('',#6852);
#742=PLANE('',#6853);
#743=PLANE('',#6854);
#744=PLANE('',#6855);
#745=PLANE('',#6857);
#746=PLANE('',#6874);
#747=PLANE('',#6893);
#748=PLANE('',#6894);
#749=PLANE('',#6895);
#918=FACE_OUTER_BOUND('',#1319,.T.);
#919=FACE_OUTER_BOUND('',#1320,.T.);
#920=FACE_OUTER_BOUND('',#1321,.T.);
#921=FACE_OUTER_BOUND('',#1322,.T.);
#922=FACE_OUTER_BOUND('',#1323,.T.);
#923=FACE_OUTER_BOUND('',#1324,.T.);
#924=FACE_OUTER_BOUND('',#1325,.T.);
#925=FACE_OUTER_BOUND('',#1326,.T.);
#926=FACE_OUTER_BOUND('',#1327,.T.);
#927=FACE_OUTER_BOUND('',#1328,.T.);
#928=FACE_OUTER_BOUND('',#1329,.T.);
#929=FACE_OUTER_BOUND('',#1331,.T.);
#930=FACE_OUTER_BOUND('',#1332,.T.);
#931=FACE_OUTER_BOUND('',#1333,.T.);
#932=FACE_OUTER_BOUND('',#1334,.T.);
#933=FACE_OUTER_BOUND('',#1335,.T.);
#934=FACE_OUTER_BOUND('',#1336,.T.);
#935=FACE_OUTER_BOUND('',#1337,.T.);
#936=FACE_OUTER_BOUND('',#1339,.T.);
#937=FACE_OUTER_BOUND('',#1340,.T.);
#938=FACE_OUTER_BOUND('',#1341,.T.);
#939=FACE_OUTER_BOUND('',#1342,.T.);
#940=FACE_OUTER_BOUND('',#1343,.T.);
#941=FACE_OUTER_BOUND('',#1344,.T.);
#942=FACE_OUTER_BOUND('',#1345,.T.);
#943=FACE_OUTER_BOUND('',#1346,.T.);
#944=FACE_OUTER_BOUND('',#1347,.T.);
#945=FACE_OUTER_BOUND('',#1348,.T.);
#946=FACE_OUTER_BOUND('',#1350,.T.);
#947=FACE_OUTER_BOUND('',#1352,.T.);
#948=FACE_OUTER_BOUND('',#1353,.T.);
#949=FACE_OUTER_BOUND('',#1354,.T.);
#950=FACE_OUTER_BOUND('',#1355,.T.);
#951=FACE_OUTER_BOUND('',#1356,.T.);
#952=FACE_OUTER_BOUND('',#1357,.T.);
#953=FACE_OUTER_BOUND('',#1358,.T.);
#954=FACE_OUTER_BOUND('',#1359,.T.);
#955=FACE_OUTER_BOUND('',#1360,.T.);
#956=FACE_OUTER_BOUND('',#1361,.T.);
#957=FACE_OUTER_BOUND('',#1362,.T.);
#958=FACE_OUTER_BOUND('',#1364,.T.);
#959=FACE_OUTER_BOUND('',#1365,.T.);
#960=FACE_OUTER_BOUND('',#1366,.T.);
#961=FACE_OUTER_BOUND('',#1367,.T.);
#962=FACE_OUTER_BOUND('',#1368,.T.);
#963=FACE_OUTER_BOUND('',#1369,.T.);
#964=FACE_OUTER_BOUND('',#1370,.T.);
#965=FACE_OUTER_BOUND('',#1371,.T.);
#966=FACE_OUTER_BOUND('',#1375,.T.);
#967=FACE_OUTER_BOUND('',#1376,.T.);
#968=FACE_OUTER_BOUND('',#1377,.T.);
#969=FACE_OUTER_BOUND('',#1378,.T.);
#970=FACE_OUTER_BOUND('',#1379,.T.);
#971=FACE_OUTER_BOUND('',#1380,.T.);
#972=FACE_OUTER_BOUND('',#1381,.T.);
#973=FACE_OUTER_BOUND('',#1382,.T.);
#974=FACE_OUTER_BOUND('',#1383,.T.);
#975=FACE_OUTER_BOUND('',#1384,.T.);
#976=FACE_OUTER_BOUND('',#1385,.T.);
#977=FACE_OUTER_BOUND('',#1386,.T.);
#978=FACE_OUTER_BOUND('',#1387,.T.);
#979=FACE_OUTER_BOUND('',#1388,.T.);
#980=FACE_OUTER_BOUND('',#1392,.T.);
#981=FACE_OUTER_BOUND('',#1393,.T.);
#982=FACE_OUTER_BOUND('',#1394,.T.);
#983=FACE_OUTER_BOUND('',#1395,.T.);
#984=FACE_OUTER_BOUND('',#1396,.T.);
#985=FACE_OUTER_BOUND('',#1397,.T.);
#986=FACE_OUTER_BOUND('',#1398,.T.);
#987=FACE_OUTER_BOUND('',#1399,.T.);
#988=FACE_OUTER_BOUND('',#1400,.T.);
#989=FACE_OUTER_BOUND('',#1401,.T.);
#990=FACE_OUTER_BOUND('',#1402,.T.);
#991=FACE_OUTER_BOUND('',#1403,.T.);
#992=FACE_OUTER_BOUND('',#1404,.T.);
#993=FACE_OUTER_BOUND('',#1405,.T.);
#994=FACE_OUTER_BOUND('',#1406,.T.);
#995=FACE_OUTER_BOUND('',#1407,.T.);
#996=FACE_OUTER_BOUND('',#1408,.T.);
#997=FACE_OUTER_BOUND('',#1409,.T.);
#998=FACE_OUTER_BOUND('',#1410,.T.);
#999=FACE_OUTER_BOUND('',#1411,.T.);
#1000=FACE_OUTER_BOUND('',#1412,.T.);
#1001=FACE_OUTER_BOUND('',#1413,.T.);
#1002=FACE_OUTER_BOUND('',#1414,.T.);
#1003=FACE_OUTER_BOUND('',#1415,.T.);
#1004=FACE_OUTER_BOUND('',#1416,.T.);
#1005=FACE_OUTER_BOUND('',#1417,.T.);
#1006=FACE_OUTER_BOUND('',#1418,.T.);
#1007=FACE_OUTER_BOUND('',#1419,.T.);
#1008=FACE_OUTER_BOUND('',#1420,.T.);
#1009=FACE_OUTER_BOUND('',#1421,.T.);
#1010=FACE_OUTER_BOUND('',#1422,.T.);
#1011=FACE_OUTER_BOUND('',#1423,.T.);
#1012=FACE_OUTER_BOUND('',#1424,.T.);
#1013=FACE_OUTER_BOUND('',#1425,.T.);
#1014=FACE_OUTER_BOUND('',#1426,.T.);
#1015=FACE_OUTER_BOUND('',#1433,.T.);
#1016=FACE_OUTER_BOUND('',#1434,.T.);
#1319=EDGE_LOOP('',(#4774,#4775,#4776,#4777));
#1320=EDGE_LOOP('',(#4778,#4779,#4780,#4781));
#1321=EDGE_LOOP('',(#4782,#4783,#4784,#4785));
#1322=EDGE_LOOP('',(#4786,#4787,#4788,#4789));
#1323=EDGE_LOOP('',(#4790,#4791,#4792,#4793));
#1324=EDGE_LOOP('',(#4794,#4795,#4796,#4797));
#1325=EDGE_LOOP('',(#4798,#4799,#4800,#4801));
#1326=EDGE_LOOP('',(#4802,#4803,#4804,#4805));
#1327=EDGE_LOOP('',(#4806,#4807,#4808,#4809));
#1328=EDGE_LOOP('',(#4810,#4811,#4812,#4813));
#1329=EDGE_LOOP('',(#4814,#4815,#4816,#4817,#4818,#4819));
#1330=EDGE_LOOP('',(#4820));
#1331=EDGE_LOOP('',(#4821,#4822,#4823,#4824));
#1332=EDGE_LOOP('',(#4825,#4826,#4827,#4828));
#1333=EDGE_LOOP('',(#4829,#4830,#4831,#4832));
#1334=EDGE_LOOP('',(#4833,#4834,#4835,#4836));
#1335=EDGE_LOOP('',(#4837,#4838,#4839,#4840));
#1336=EDGE_LOOP('',(#4841,#4842,#4843,#4844));
#1337=EDGE_LOOP('',(#4845,#4846,#4847,#4848,#4849,#4850));
#1338=EDGE_LOOP('',(#4851));
#1339=EDGE_LOOP('',(#4852,#4853,#4854,#4855));
#1340=EDGE_LOOP('',(#4856,#4857,#4858,#4859));
#1341=EDGE_LOOP('',(#4860,#4861,#4862,#4863));
#1342=EDGE_LOOP('',(#4864,#4865,#4866,#4867));
#1343=EDGE_LOOP('',(#4868,#4869,#4870,#4871));
#1344=EDGE_LOOP('',(#4872,#4873,#4874,#4875));
#1345=EDGE_LOOP('',(#4876,#4877,#4878,#4879));
#1346=EDGE_LOOP('',(#4880,#4881,#4882,#4883));
#1347=EDGE_LOOP('',(#4884,#4885,#4886,#4887));
#1348=EDGE_LOOP('',(#4888));
#1349=EDGE_LOOP('',(#4889));
#1350=EDGE_LOOP('',(#4890));
#1351=EDGE_LOOP('',(#4891));
#1352=EDGE_LOOP('',(#4892,#4893,#4894,#4895));
#1353=EDGE_LOOP('',(#4896,#4897,#4898,#4899));
#1354=EDGE_LOOP('',(#4900,#4901,#4902,#4903));
#1355=EDGE_LOOP('',(#4904,#4905,#4906,#4907));
#1356=EDGE_LOOP('',(#4908,#4909,#4910,#4911));
#1357=EDGE_LOOP('',(#4912,#4913,#4914,#4915,#4916,#4917));
#1358=EDGE_LOOP('',(#4918,#4919,#4920,#4921,#4922,#4923,#4924,#4925,#4926,
#4927));
#1359=EDGE_LOOP('',(#4928,#4929,#4930,#4931,#4932,#4933,#4934,#4935,#4936,
#4937));
#1360=EDGE_LOOP('',(#4938,#4939,#4940,#4941,#4942,#4943,#4944,#4945,#4946,
#4947));
#1361=EDGE_LOOP('',(#4948,#4949,#4950,#4951,#4952,#4953,#4954,#4955));
#1362=EDGE_LOOP('',(#4956,#4957,#4958,#4959,#4960,#4961,#4962,#4963,#4964,
#4965,#4966,#4967,#4968,#4969,#4970,#4971,#4972,#4973,#4974,#4975,#4976,
#4977,#4978,#4979,#4980,#4981,#4982,#4983,#4984,#4985,#4986,#4987,#4988,
#4989,#4990,#4991,#4992,#4993,#4994,#4995,#4996,#4997));
#1363=EDGE_LOOP('',(#4998,#4999,#5000,#5001,#5002,#5003));
#1364=EDGE_LOOP('',(#5004,#5005,#5006,#5007));
#1365=EDGE_LOOP('',(#5008,#5009,#5010,#5011));
#1366=EDGE_LOOP('',(#5012,#5013,#5014,#5015,#5016,#5017));
#1367=EDGE_LOOP('',(#5018,#5019,#5020,#5021));
#1368=EDGE_LOOP('',(#5022,#5023,#5024,#5025));
#1369=EDGE_LOOP('',(#5026,#5027,#5028,#5029));
#1370=EDGE_LOOP('',(#5030,#5031,#5032,#5033));
#1371=EDGE_LOOP('',(#5034,#5035,#5036,#5037));
#1372=EDGE_LOOP('',(#5038));
#1373=EDGE_LOOP('',(#5039));
#1374=EDGE_LOOP('',(#5040));
#1375=EDGE_LOOP('',(#5041,#5042,#5043,#5044));
#1376=EDGE_LOOP('',(#5045,#5046,#5047,#5048));
#1377=EDGE_LOOP('',(#5049,#5050,#5051,#5052));
#1378=EDGE_LOOP('',(#5053,#5054,#5055,#5056));
#1379=EDGE_LOOP('',(#5057,#5058,#5059,#5060,#5061,#5062,#5063,#5064,#5065,
#5066));
#1380=EDGE_LOOP('',(#5067,#5068,#5069,#5070));
#1381=EDGE_LOOP('',(#5071,#5072,#5073,#5074));
#1382=EDGE_LOOP('',(#5075,#5076,#5077,#5078));
#1383=EDGE_LOOP('',(#5079,#5080,#5081,#5082));
#1384=EDGE_LOOP('',(#5083,#5084,#5085,#5086));
#1385=EDGE_LOOP('',(#5087,#5088,#5089,#5090,#5091,#5092,#5093,#5094,#5095,
#5096));
#1386=EDGE_LOOP('',(#5097,#5098,#5099,#5100));
#1387=EDGE_LOOP('',(#5101,#5102,#5103,#5104));
#1388=EDGE_LOOP('',(#5105,#5106,#5107,#5108));
#1389=EDGE_LOOP('',(#5109));
#1390=EDGE_LOOP('',(#5110));
#1391=EDGE_LOOP('',(#5111));
#1392=EDGE_LOOP('',(#5112,#5113,#5114,#5115));
#1393=EDGE_LOOP('',(#5116,#5117,#5118,#5119));
#1394=EDGE_LOOP('',(#5120,#5121,#5122,#5123,#5124,#5125,#5126,#5127,#5128,
#5129));
#1395=EDGE_LOOP('',(#5130,#5131,#5132,#5133));
#1396=EDGE_LOOP('',(#5134,#5135,#5136,#5137));
#1397=EDGE_LOOP('',(#5138,#5139,#5140,#5141));
#1398=EDGE_LOOP('',(#5142,#5143,#5144,#5145));
#1399=EDGE_LOOP('',(#5146,#5147,#5148,#5149));
#1400=EDGE_LOOP('',(#5150,#5151,#5152));
#1401=EDGE_LOOP('',(#5153,#5154,#5155));
#1402=EDGE_LOOP('',(#5156,#5157,#5158));
#1403=EDGE_LOOP('',(#5159,#5160,#5161,#5162));
#1404=EDGE_LOOP('',(#5163,#5164,#5165,#5166));
#1405=EDGE_LOOP('',(#5167,#5168,#5169));
#1406=EDGE_LOOP('',(#5170,#5171,#5172,#5173));
#1407=EDGE_LOOP('',(#5174,#5175,#5176,#5177));
#1408=EDGE_LOOP('',(#5178,#5179,#5180,#5181));
#1409=EDGE_LOOP('',(#5182,#5183,#5184,#5185));
#1410=EDGE_LOOP('',(#5186,#5187,#5188,#5189));
#1411=EDGE_LOOP('',(#5190,#5191,#5192,#5193));
#1412=EDGE_LOOP('',(#5194,#5195,#5196));
#1413=EDGE_LOOP('',(#5197,#5198,#5199));
#1414=EDGE_LOOP('',(#5200,#5201,#5202));
#1415=EDGE_LOOP('',(#5203,#5204,#5205,#5206));
#1416=EDGE_LOOP('',(#5207,#5208,#5209,#5210));
#1417=EDGE_LOOP('',(#5211,#5212,#5213));
#1418=EDGE_LOOP('',(#5214,#5215,#5216,#5217));
#1419=EDGE_LOOP('',(#5218,#5219,#5220,#5221));
#1420=EDGE_LOOP('',(#5222,#5223,#5224,#5225));
#1421=EDGE_LOOP('',(#5226,#5227,#5228,#5229));
#1422=EDGE_LOOP('',(#5230,#5231,#5232,#5233));
#1423=EDGE_LOOP('',(#5234,#5235,#5236,#5237));
#1424=EDGE_LOOP('',(#5238,#5239,#5240,#5241));
#1425=EDGE_LOOP('',(#5242,#5243,#5244,#5245,#5246,#5247,#5248,#5249));
#1426=EDGE_LOOP('',(#5250,#5251,#5252,#5253));
#1427=EDGE_LOOP('',(#5254,#5255,#5256,#5257,#5258,#5259));
#1428=EDGE_LOOP('',(#5260,#5261,#5262,#5263,#5264,#5265));
#1429=EDGE_LOOP('',(#5266));
#1430=EDGE_LOOP('',(#5267));
#1431=EDGE_LOOP('',(#5268));
#1432=EDGE_LOOP('',(#5269));
#1433=EDGE_LOOP('',(#5270,#5271,#5272,#5273));
#1434=EDGE_LOOP('',(#5274,#5275,#5276,#5277));
#1749=LINE('',#10636,#2153);
#1750=LINE('',#10642,#2154);
#1751=LINE('',#10648,#2155);
#1752=LINE('',#10654,#2156);
#1753=LINE('',#10659,#2157);
#1754=LINE('',#10661,#2158);
#1755=LINE('',#10663,#2159);
#1756=LINE('',#10664,#2160);
#1757=LINE('',#10667,#2161);
#1758=LINE('',#10669,#2162);
#1759=LINE('',#10670,#2163);
#1760=LINE('',#10673,#2164);
#1761=LINE('',#10675,#2165);
#1762=LINE('',#10676,#2166);
#1763=LINE('',#10679,#2167);
#1764=LINE('',#10681,#2168);
#1765=LINE('',#10682,#2169);
#1766=LINE('',#10685,#2170);
#1767=LINE('',#10687,#2171);
#1768=LINE('',#10688,#2172);
#1769=LINE('',#10690,#2173);
#1770=LINE('',#10691,#2174);
#1771=LINE('',#10698,#2175);
#1772=LINE('',#10700,#2176);
#1773=LINE('',#10702,#2177);
#1774=LINE('',#10703,#2178);
#1775=LINE('',#10706,#2179);
#1776=LINE('',#10708,#2180);
#1777=LINE('',#10709,#2181);
#1778=LINE('',#10712,#2182);
#1779=LINE('',#10714,#2183);
#1780=LINE('',#10715,#2184);
#1781=LINE('',#10718,#2185);
#1782=LINE('',#10720,#2186);
#1783=LINE('',#10721,#2187);
#1784=LINE('',#10724,#2188);
#1785=LINE('',#10726,#2189);
#1786=LINE('',#10727,#2190);
#1787=LINE('',#10729,#2191);
#1788=LINE('',#10730,#2192);
#1789=LINE('',#10736,#2193);
#1790=LINE('',#10740,#2194);
#1791=LINE('',#10745,#2195);
#1792=LINE('',#10747,#2196);
#1793=LINE('',#10749,#2197);
#1794=LINE('',#10750,#2198);
#1795=LINE('',#10754,#2199);
#1796=LINE('',#10756,#2200);
#1797=LINE('',#10758,#2201);
#1798=LINE('',#10759,#2202);
#1799=LINE('',#10763,#2203);
#1800=LINE('',#10765,#2204);
#1801=LINE('',#10767,#2205);
#1802=LINE('',#10768,#2206);
#1803=LINE('',#10772,#2207);
#1804=LINE('',#10774,#2208);
#1805=LINE('',#10776,#2209);
#1806=LINE('',#10777,#2210);
#1807=LINE('',#10781,#2211);
#1808=LINE('',#10783,#2212);
#1809=LINE('',#10785,#2213);
#1810=LINE('',#10786,#2214);
#1811=LINE('',#10790,#2215);
#1812=LINE('',#10792,#2216);
#1813=LINE('',#10794,#2217);
#1814=LINE('',#10795,#2218);
#1815=LINE('',#10799,#2219);
#1816=LINE('',#10801,#2220);
#1817=LINE('',#10803,#2221);
#1818=LINE('',#10804,#2222);
#1819=LINE('',#10812,#2223);
#1820=LINE('',#10813,#2224);
#1821=LINE('',#10815,#2225);
#1822=LINE('',#10816,#2226);
#1823=LINE('',#10818,#2227);
#1824=LINE('',#10819,#2228);
#1825=LINE('',#10822,#2229);
#1826=LINE('',#10824,#2230);
#1827=LINE('',#10825,#2231);
#1828=LINE('',#10828,#2232);
#1829=LINE('',#10830,#2233);
#1830=LINE('',#10831,#2234);
#1831=LINE('',#10835,#2235);
#1832=LINE('',#10873,#2236);
#1833=LINE('',#10911,#2237);
#1834=LINE('',#10949,#2238);
#1835=LINE('',#10986,#2239);
#1836=LINE('',#10989,#2240);
#1837=LINE('',#11027,#2241);
#1838=LINE('',#11064,#2242);
#1839=LINE('',#11067,#2243);
#1840=LINE('',#11105,#2244);
#1841=LINE('',#11142,#2245);
#1842=LINE('',#11145,#2246);
#1843=LINE('',#11152,#2247);
#1844=LINE('',#11158,#2248);
#1845=LINE('',#11175,#2249);
#1846=LINE('',#11184,#2250);
#1847=LINE('',#11190,#2251);
#1848=LINE('',#11225,#2252);
#1849=LINE('',#11296,#2253);
#1850=LINE('',#11366,#2254);
#1851=LINE('',#11401,#2255);
#1852=LINE('',#11407,#2256);
#1853=LINE('',#11416,#2257);
#1854=LINE('',#11450,#2258);
#1855=LINE('',#11482,#2259);
#1856=LINE('',#11486,#2260);
#1857=LINE('',#11490,#2261);
#1858=LINE('',#11536,#2262);
#1859=LINE('',#11671,#2263);
#1860=LINE('',#11775,#2264);
#1861=LINE('',#11938,#2265);
#1862=LINE('',#12101,#2266);
#1863=LINE('',#12190,#2267);
#1864=LINE('',#12278,#2268);
#1865=LINE('',#12390,#2269);
#1866=LINE('',#12391,#2270);
#1867=LINE('',#12428,#2271);
#1868=LINE('',#12429,#2272);
#2153=VECTOR('',#7632,0.15);
#2154=VECTOR('',#7639,0.15);
#2155=VECTOR('',#7646,0.15);
#2156=VECTOR('',#7653,0.15);
#2157=VECTOR('',#7658,1.);
#2158=VECTOR('',#7659,1.);
#2159=VECTOR('',#7660,1.);
#2160=VECTOR('',#7661,1.);
#2161=VECTOR('',#7664,1.);
#2162=VECTOR('',#7665,1.);
#2163=VECTOR('',#7666,1.);
#2164=VECTOR('',#7669,1.);
#2165=VECTOR('',#7670,1.);
#2166=VECTOR('',#7671,1.);
#2167=VECTOR('',#7674,1.);
#2168=VECTOR('',#7675,1.);
#2169=VECTOR('',#7676,1.);
#2170=VECTOR('',#7679,1.);
#2171=VECTOR('',#7680,1.);
#2172=VECTOR('',#7681,1.);
#2173=VECTOR('',#7684,1.);
#2174=VECTOR('',#7685,1.);
#2175=VECTOR('',#7692,1.);
#2176=VECTOR('',#7693,1.);
#2177=VECTOR('',#7694,1.);
#2178=VECTOR('',#7695,1.);
#2179=VECTOR('',#7698,1.);
#2180=VECTOR('',#7699,1.);
#2181=VECTOR('',#7700,1.);
#2182=VECTOR('',#7703,1.);
#2183=VECTOR('',#7704,1.);
#2184=VECTOR('',#7705,1.);
#2185=VECTOR('',#7708,1.);
#2186=VECTOR('',#7709,1.);
#2187=VECTOR('',#7710,1.);
#2188=VECTOR('',#7713,1.);
#2189=VECTOR('',#7714,1.);
#2190=VECTOR('',#7715,1.);
#2191=VECTOR('',#7718,1.);
#2192=VECTOR('',#7719,1.);
#2193=VECTOR('',#7726,0.17);
#2194=VECTOR('',#7731,0.17);
#2195=VECTOR('',#7736,1.);
#2196=VECTOR('',#7737,1.);
#2197=VECTOR('',#7738,1.);
#2198=VECTOR('',#7739,1.);
#2199=VECTOR('',#7742,1.);
#2200=VECTOR('',#7743,1.);
#2201=VECTOR('',#7744,1.);
#2202=VECTOR('',#7745,1.);
#2203=VECTOR('',#7748,1.);
#2204=VECTOR('',#7749,1.);
#2205=VECTOR('',#7750,1.);
#2206=VECTOR('',#7751,1.);
#2207=VECTOR('',#7754,1.);
#2208=VECTOR('',#7755,1.);
#2209=VECTOR('',#7756,1.);
#2210=VECTOR('',#7757,1.);
#2211=VECTOR('',#7760,1.);
#2212=VECTOR('',#7761,1.);
#2213=VECTOR('',#7762,1.);
#2214=VECTOR('',#7763,1.);
#2215=VECTOR('',#7766,1.);
#2216=VECTOR('',#7767,1.);
#2217=VECTOR('',#7768,1.);
#2218=VECTOR('',#7769,1.);
#2219=VECTOR('',#7772,1.);
#2220=VECTOR('',#7773,1.);
#2221=VECTOR('',#7774,1.);
#2222=VECTOR('',#7775,1.);
#2223=VECTOR('',#7786,1.);
#2224=VECTOR('',#7787,1.);
#2225=VECTOR('',#7790,1.);
#2226=VECTOR('',#7791,1.);
#2227=VECTOR('',#7794,1.);
#2228=VECTOR('',#7795,1.);
#2229=VECTOR('',#7798,1.);
#2230=VECTOR('',#7799,1.);
#2231=VECTOR('',#7800,1.);
#2232=VECTOR('',#7803,1.);
#2233=VECTOR('',#7804,1.);
#2234=VECTOR('',#7805,1.);
#2235=VECTOR('',#7808,1.);
#2236=VECTOR('',#7809,1.);
#2237=VECTOR('',#7812,1.);
#2238=VECTOR('',#7813,1.);
#2239=VECTOR('',#7814,1.);
#2240=VECTOR('',#7817,1.);
#2241=VECTOR('',#7818,1.);
#2242=VECTOR('',#7819,1.);
#2243=VECTOR('',#7822,1.);
#2244=VECTOR('',#7823,1.);
#2245=VECTOR('',#7824,1.);
#2246=VECTOR('',#7827,1.);
#2247=VECTOR('',#7828,1.);
#2248=VECTOR('',#7829,1.);
#2249=VECTOR('',#7832,1.);
#2250=VECTOR('',#7833,1.);
#2251=VECTOR('',#7834,1.);
#2252=VECTOR('',#7835,1.);
#2253=VECTOR('',#7836,1.);
#2254=VECTOR('',#7837,1.);
#2255=VECTOR('',#7838,1.);
#2256=VECTOR('',#7839,1.);
#2257=VECTOR('',#7840,1.);
#2258=VECTOR('',#7841,1.);
#2259=VECTOR('',#7842,1.);
#2260=VECTOR('',#7847,0.4);
#2261=VECTOR('',#7852,0.4);
#2262=VECTOR('',#7855,1.);
#2263=VECTOR('',#7862,1.);
#2264=VECTOR('',#7865,1.);
#2265=VECTOR('',#7870,1.);
#2266=VECTOR('',#7875,1.);
#2267=VECTOR('',#7880,1.);
#2268=VECTOR('',#7913,1.);
#2269=VECTOR('',#7942,1.);
#2270=VECTOR('',#7943,1.);
#2271=VECTOR('',#7954,1.);
#2272=VECTOR('',#7955,1.);
#2482=CIRCLE('',#6790,0.15);
#2483=CIRCLE('',#6791,0.15);
#2484=CIRCLE('',#6793,0.15);
#2485=CIRCLE('',#6794,0.15);
#2486=CIRCLE('',#6796,0.15);
#2487=CIRCLE('',#6797,0.15);
#2488=CIRCLE('',#6799,0.15);
#2489=CIRCLE('',#6800,0.15);
#2490=CIRCLE('',#6808,0.17);
#2491=CIRCLE('',#6816,0.17);
#2492=CIRCLE('',#6818,0.17);
#2493=CIRCLE('',#6820,0.17);
#2494=CIRCLE('',#6829,0.4);
#2495=CIRCLE('',#6831,0.4);
#2496=CIRCLE('',#6844,0.4);
#2497=CIRCLE('',#6846,0.4);
#2498=CIRCLE('',#6848,0.1);
#2499=CIRCLE('',#6856,0.0999999999999994);
#2500=CIRCLE('',#6858,0.0999999999999999);
#2501=CIRCLE('',#6860,0.1);
#2502=CIRCLE('',#6861,0.1);
#2503=CIRCLE('',#6863,0.100000000000001);
#2504=CIRCLE('',#6864,0.100000000000001);
#2505=CIRCLE('',#6865,0.100000000000002);
#2506=CIRCLE('',#6867,0.0999999999999995);
#2507=CIRCLE('',#6868,0.0999999999999991);
#2508=CIRCLE('',#6871,0.100000000000001);
#2509=CIRCLE('',#6872,0.1);
#2510=CIRCLE('',#6876,0.3);
#2511=CIRCLE('',#6877,0.3);
#2512=CIRCLE('',#6878,0.3);
#2513=CIRCLE('',#6880,0.3);
#2514=CIRCLE('',#6881,0.300000000000002);
#2515=CIRCLE('',#6882,0.3);
#2516=CIRCLE('',#6884,0.3);
#2517=CIRCLE('',#6885,0.299999999999999);
#2518=CIRCLE('',#6886,0.3);
#2519=CIRCLE('',#6889,0.300000000000001);
#2520=CIRCLE('',#6890,0.3);
#2521=CIRCLE('',#6891,0.3);
#2779=VERTEX_POINT('',#10633);
#2780=VERTEX_POINT('',#10635);
#2781=VERTEX_POINT('',#10639);
#2782=VERTEX_POINT('',#10641);
#2783=VERTEX_POINT('',#10645);
#2784=VERTEX_POINT('',#10647);
#2785=VERTEX_POINT('',#10651);
#2786=VERTEX_POINT('',#10653);
#2787=VERTEX_POINT('',#10657);
#2788=VERTEX_POINT('',#10658);
#2789=VERTEX_POINT('',#10660);
#2790=VERTEX_POINT('',#10662);
#2791=VERTEX_POINT('',#10666);
#2792=VERTEX_POINT('',#10668);
#2793=VERTEX_POINT('',#10672);
#2794=VERTEX_POINT('',#10674);
#2795=VERTEX_POINT('',#10678);
#2796=VERTEX_POINT('',#10680);
#2797=VERTEX_POINT('',#10684);
#2798=VERTEX_POINT('',#10686);
#2799=VERTEX_POINT('',#10693);
#2800=VERTEX_POINT('',#10696);
#2801=VERTEX_POINT('',#10697);
#2802=VERTEX_POINT('',#10699);
#2803=VERTEX_POINT('',#10701);
#2804=VERTEX_POINT('',#10705);
#2805=VERTEX_POINT('',#10707);
#2806=VERTEX_POINT('',#10711);
#2807=VERTEX_POINT('',#10713);
#2808=VERTEX_POINT('',#10717);
#2809=VERTEX_POINT('',#10719);
#2810=VERTEX_POINT('',#10723);
#2811=VERTEX_POINT('',#10725);
#2812=VERTEX_POINT('',#10732);
#2813=VERTEX_POINT('',#10735);
#2814=VERTEX_POINT('',#10739);
#2815=VERTEX_POINT('',#10743);
#2816=VERTEX_POINT('',#10744);
#2817=VERTEX_POINT('',#10746);
#2818=VERTEX_POINT('',#10748);
#2819=VERTEX_POINT('',#10752);
#2820=VERTEX_POINT('',#10753);
#2821=VERTEX_POINT('',#10755);
#2822=VERTEX_POINT('',#10757);
#2823=VERTEX_POINT('',#10761);
#2824=VERTEX_POINT('',#10762);
#2825=VERTEX_POINT('',#10764);
#2826=VERTEX_POINT('',#10766);
#2827=VERTEX_POINT('',#10770);
#2828=VERTEX_POINT('',#10771);
#2829=VERTEX_POINT('',#10773);
#2830=VERTEX_POINT('',#10775);
#2831=VERTEX_POINT('',#10779);
#2832=VERTEX_POINT('',#10780);
#2833=VERTEX_POINT('',#10782);
#2834=VERTEX_POINT('',#10784);
#2835=VERTEX_POINT('',#10788);
#2836=VERTEX_POINT('',#10789);
#2837=VERTEX_POINT('',#10791);
#2838=VERTEX_POINT('',#10793);
#2839=VERTEX_POINT('',#10797);
#2840=VERTEX_POINT('',#10798);
#2841=VERTEX_POINT('',#10800);
#2842=VERTEX_POINT('',#10802);
#2843=VERTEX_POINT('',#10806);
#2844=VERTEX_POINT('',#10809);
#2845=VERTEX_POINT('',#10821);
#2846=VERTEX_POINT('',#10823);
#2847=VERTEX_POINT('',#10827);
#2848=VERTEX_POINT('',#10829);
#2849=VERTEX_POINT('',#10833);
#2850=VERTEX_POINT('',#10834);
#2851=VERTEX_POINT('',#10836);
#2852=VERTEX_POINT('',#10843);
#2853=VERTEX_POINT('',#10872);
#2854=VERTEX_POINT('',#10874);
#2855=VERTEX_POINT('',#10910);
#2856=VERTEX_POINT('',#10912);
#2857=VERTEX_POINT('',#10919);
#2858=VERTEX_POINT('',#10948);
#2859=VERTEX_POINT('',#10950);
#2860=VERTEX_POINT('',#10979);
#2861=VERTEX_POINT('',#10988);
#2862=VERTEX_POINT('',#10990);
#2863=VERTEX_POINT('',#10997);
#2864=VERTEX_POINT('',#11026);
#2865=VERTEX_POINT('',#11028);
#2866=VERTEX_POINT('',#11057);
#2867=VERTEX_POINT('',#11066);
#2868=VERTEX_POINT('',#11068);
#2869=VERTEX_POINT('',#11075);
#2870=VERTEX_POINT('',#11104);
#2871=VERTEX_POINT('',#11106);
#2872=VERTEX_POINT('',#11135);
#2873=VERTEX_POINT('',#11144);
#2874=VERTEX_POINT('',#11146);
#2875=VERTEX_POINT('',#11151);
#2876=VERTEX_POINT('',#11153);
#2877=VERTEX_POINT('',#11174);
#2878=VERTEX_POINT('',#11183);
#2879=VERTEX_POINT('',#11189);
#2880=VERTEX_POINT('',#11191);
#2881=VERTEX_POINT('',#11224);
#2882=VERTEX_POINT('',#11226);
#2883=VERTEX_POINT('',#11258);
#2884=VERTEX_POINT('',#11263);
#2885=VERTEX_POINT('',#11295);
#2886=VERTEX_POINT('',#11297);
#2887=VERTEX_POINT('',#11329);
#2888=VERTEX_POINT('',#11334);
#2889=VERTEX_POINT('',#11367);
#2890=VERTEX_POINT('',#11396);
#2891=VERTEX_POINT('',#11402);
#2892=VERTEX_POINT('',#11408);
#2893=VERTEX_POINT('',#11417);
#2894=VERTEX_POINT('',#11418);
#2895=VERTEX_POINT('',#11423);
#2896=VERTEX_POINT('',#11449);
#2897=VERTEX_POINT('',#11451);
#2898=VERTEX_POINT('',#11477);
#2899=VERTEX_POINT('',#11484);
#2900=VERTEX_POINT('',#11488);
#2901=VERTEX_POINT('',#11492);
#2902=VERTEX_POINT('',#11499);
#2903=VERTEX_POINT('',#11506);
#2904=VERTEX_POINT('',#11535);
#2905=VERTEX_POINT('',#11601);
#2906=VERTEX_POINT('',#11654);
#2907=VERTEX_POINT('',#11666);
#2908=VERTEX_POINT('',#11728);
#2909=VERTEX_POINT('',#11738);
#2910=VERTEX_POINT('',#11745);
#2911=VERTEX_POINT('',#11774);
#2912=VERTEX_POINT('',#11776);
#2913=VERTEX_POINT('',#11901);
#2914=VERTEX_POINT('',#11908);
#2915=VERTEX_POINT('',#11937);
#2916=VERTEX_POINT('',#11939);
#2917=VERTEX_POINT('',#12064);
#2918=VERTEX_POINT('',#12071);
#2919=VERTEX_POINT('',#12100);
#2920=VERTEX_POINT('',#12102);
#2921=VERTEX_POINT('',#12153);
#2922=VERTEX_POINT('',#12182);
#2923=VERTEX_POINT('',#12189);
#2924=VERTEX_POINT('',#12211);
#2925=VERTEX_POINT('',#12246);
#2926=VERTEX_POINT('',#12274);
#2927=VERTEX_POINT('',#12369);
#2928=VERTEX_POINT('',#12370);
#2929=VERTEX_POINT('',#12372);
#2930=VERTEX_POINT('',#12376);
#2931=VERTEX_POINT('',#12377);
#2932=VERTEX_POINT('',#12379);
#2933=VERTEX_POINT('',#12383);
#2934=VERTEX_POINT('',#12384);
#2935=VERTEX_POINT('',#12386);
#2936=VERTEX_POINT('',#12421);
#2937=VERTEX_POINT('',#12422);
#2938=VERTEX_POINT('',#12424);
#3504=EDGE_CURVE('',#2779,#2779,#2482,.T.);
#3505=EDGE_CURVE('',#2779,#2780,#1749,.T.);
#3506=EDGE_CURVE('',#2780,#2780,#2483,.T.);
#3507=EDGE_CURVE('',#2781,#2781,#2484,.T.);
#3508=EDGE_CURVE('',#2781,#2782,#1750,.T.);
#3509=EDGE_CURVE('',#2782,#2782,#2485,.T.);
#3510=EDGE_CURVE('',#2783,#2783,#2486,.T.);
#3511=EDGE_CURVE('',#2783,#2784,#1751,.T.);
#3512=EDGE_CURVE('',#2784,#2784,#2487,.T.);
#3513=EDGE_CURVE('',#2785,#2785,#2488,.T.);
#3514=EDGE_CURVE('',#2785,#2786,#1752,.T.);
#3515=EDGE_CURVE('',#2786,#2786,#2489,.T.);
#3516=EDGE_CURVE('',#2787,#2788,#1753,.T.);
#3517=EDGE_CURVE('',#2787,#2789,#1754,.T.);
#3518=EDGE_CURVE('',#2789,#2790,#1755,.T.);
#3519=EDGE_CURVE('',#2788,#2790,#1756,.T.);
#3520=EDGE_CURVE('',#2791,#2787,#1757,.T.);
#3521=EDGE_CURVE('',#2791,#2792,#1758,.T.);
#3522=EDGE_CURVE('',#2792,#2789,#1759,.T.);
#3523=EDGE_CURVE('',#2793,#2791,#1760,.T.);
#3524=EDGE_CURVE('',#2793,#2794,#1761,.T.);
#3525=EDGE_CURVE('',#2794,#2792,#1762,.T.);
#3526=EDGE_CURVE('',#2795,#2793,#1763,.T.);
#3527=EDGE_CURVE('',#2795,#2796,#1764,.T.);
#3528=EDGE_CURVE('',#2796,#2794,#1765,.T.);
#3529=EDGE_CURVE('',#2797,#2795,#1766,.T.);
#3530=EDGE_CURVE('',#2797,#2798,#1767,.T.);
#3531=EDGE_CURVE('',#2798,#2796,#1768,.T.);
#3532=EDGE_CURVE('',#2788,#2797,#1769,.T.);
#3533=EDGE_CURVE('',#2790,#2798,#1770,.T.);
#3534=EDGE_CURVE('',#2799,#2799,#2490,.T.);
#3535=EDGE_CURVE('',#2800,#2801,#1771,.T.);
#3536=EDGE_CURVE('',#2800,#2802,#1772,.T.);
#3537=EDGE_CURVE('',#2802,#2803,#1773,.T.);
#3538=EDGE_CURVE('',#2801,#2803,#1774,.T.);
#3539=EDGE_CURVE('',#2804,#2800,#1775,.T.);
#3540=EDGE_CURVE('',#2804,#2805,#1776,.T.);
#3541=EDGE_CURVE('',#2805,#2802,#1777,.T.);
#3542=EDGE_CURVE('',#2806,#2804,#1778,.T.);
#3543=EDGE_CURVE('',#2806,#2807,#1779,.T.);
#3544=EDGE_CURVE('',#2807,#2805,#1780,.T.);
#3545=EDGE_CURVE('',#2808,#2806,#1781,.T.);
#3546=EDGE_CURVE('',#2808,#2809,#1782,.T.);
#3547=EDGE_CURVE('',#2809,#2807,#1783,.T.);
#3548=EDGE_CURVE('',#2810,#2808,#1784,.T.);
#3549=EDGE_CURVE('',#2810,#2811,#1785,.T.);
#3550=EDGE_CURVE('',#2811,#2809,#1786,.T.);
#3551=EDGE_CURVE('',#2801,#2810,#1787,.T.);
#3552=EDGE_CURVE('',#2803,#2811,#1788,.T.);
#3553=EDGE_CURVE('',#2812,#2812,#2491,.T.);
#3554=EDGE_CURVE('',#2812,#2813,#1789,.T.);
#3555=EDGE_CURVE('',#2813,#2813,#2492,.T.);
#3556=EDGE_CURVE('',#2799,#2814,#1790,.T.);
#3557=EDGE_CURVE('',#2814,#2814,#2493,.T.);
#3558=EDGE_CURVE('',#2815,#2816,#1791,.T.);
#3559=EDGE_CURVE('',#2817,#2815,#1792,.T.);
#3560=EDGE_CURVE('',#2818,#2817,#1793,.T.);
#3561=EDGE_CURVE('',#2818,#2816,#1794,.T.);
#3562=EDGE_CURVE('',#2819,#2820,#1795,.T.);
#3563=EDGE_CURVE('',#2819,#2821,#1796,.T.);
#3564=EDGE_CURVE('',#2822,#2821,#1797,.T.);
#3565=EDGE_CURVE('',#2820,#2822,#1798,.T.);
#3566=EDGE_CURVE('',#2823,#2824,#1799,.T.);
#3567=EDGE_CURVE('',#2823,#2825,#1800,.T.);
#3568=EDGE_CURVE('',#2826,#2825,#1801,.T.);
#3569=EDGE_CURVE('',#2824,#2826,#1802,.T.);
#3570=EDGE_CURVE('',#2827,#2828,#1803,.T.);
#3571=EDGE_CURVE('',#2827,#2829,#1804,.T.);
#3572=EDGE_CURVE('',#2830,#2829,#1805,.T.);
#3573=EDGE_CURVE('',#2828,#2830,#1806,.T.);
#3574=EDGE_CURVE('',#2831,#2832,#1807,.T.);
#3575=EDGE_CURVE('',#2831,#2833,#1808,.T.);
#3576=EDGE_CURVE('',#2834,#2833,#1809,.T.);
#3577=EDGE_CURVE('',#2832,#2834,#1810,.T.);
#3578=EDGE_CURVE('',#2835,#2836,#1811,.T.);
#3579=EDGE_CURVE('',#2837,#2835,#1812,.T.);
#3580=EDGE_CURVE('',#2838,#2837,#1813,.T.);
#3581=EDGE_CURVE('',#2838,#2836,#1814,.T.);
#3582=EDGE_CURVE('',#2839,#2840,#1815,.T.);
#3583=EDGE_CURVE('',#2841,#2839,#1816,.T.);
#3584=EDGE_CURVE('',#2842,#2841,#1817,.T.);
#3585=EDGE_CURVE('',#2842,#2840,#1818,.T.);
#3586=EDGE_CURVE('',#2843,#2843,#2494,.T.);
#3587=EDGE_CURVE('',#2844,#2844,#2495,.T.);
#3588=EDGE_CURVE('',#2816,#2831,#1819,.T.);
#3589=EDGE_CURVE('',#2833,#2818,#1820,.T.);
#3590=EDGE_CURVE('',#2836,#2819,#1821,.T.);
#3591=EDGE_CURVE('',#2821,#2838,#1822,.T.);
#3592=EDGE_CURVE('',#2840,#2823,#1823,.T.);
#3593=EDGE_CURVE('',#2825,#2842,#1824,.T.);
#3594=EDGE_CURVE('',#2845,#2827,#1825,.T.);
#3595=EDGE_CURVE('',#2846,#2845,#1826,.T.);
#3596=EDGE_CURVE('',#2829,#2846,#1827,.T.);
#3597=EDGE_CURVE('',#2847,#2845,#1828,.T.);
#3598=EDGE_CURVE('',#2848,#2847,#1829,.T.);
#3599=EDGE_CURVE('',#2846,#2848,#1830,.T.);
#3600=EDGE_CURVE('',#2849,#2850,#1831,.T.);
#3601=EDGE_CURVE('',#2851,#2850,#263,.T.);
#3602=EDGE_CURVE('',#2852,#2851,#264,.T.);
#3603=EDGE_CURVE('',#2853,#2852,#1832,.T.);
#3604=EDGE_CURVE('',#2854,#2853,#265,.T.);
#3605=EDGE_CURVE('',#2849,#2854,#266,.T.);
#3606=EDGE_CURVE('',#2848,#2855,#1833,.T.);
#3607=EDGE_CURVE('',#2856,#2855,#267,.T.);
#3608=EDGE_CURVE('',#2857,#2856,#268,.T.);
#3609=EDGE_CURVE('',#2858,#2857,#1834,.T.);
#3610=EDGE_CURVE('',#2859,#2858,#269,.T.);
#3611=EDGE_CURVE('',#2860,#2859,#270,.T.);
#3612=EDGE_CURVE('',#2860,#2830,#1835,.T.);
#3613=EDGE_CURVE('',#2841,#2861,#1836,.T.);
#3614=EDGE_CURVE('',#2862,#2861,#271,.T.);
#3615=EDGE_CURVE('',#2863,#2862,#272,.T.);
#3616=EDGE_CURVE('',#2864,#2863,#1837,.T.);
#3617=EDGE_CURVE('',#2865,#2864,#273,.T.);
#3618=EDGE_CURVE('',#2866,#2865,#274,.T.);
#3619=EDGE_CURVE('',#2866,#2826,#1838,.T.);
#3620=EDGE_CURVE('',#2837,#2867,#1839,.T.);
#3621=EDGE_CURVE('',#2868,#2867,#275,.T.);
#3622=EDGE_CURVE('',#2869,#2868,#276,.T.);
#3623=EDGE_CURVE('',#2870,#2869,#1840,.T.);
#3624=EDGE_CURVE('',#2871,#2870,#277,.T.);
#3625=EDGE_CURVE('',#2872,#2871,#278,.T.);
#3626=EDGE_CURVE('',#2872,#2822,#1841,.T.);
#3627=EDGE_CURVE('',#2873,#2832,#1842,.T.);
#3628=EDGE_CURVE('',#2873,#2874,#279,.T.);
#3629=EDGE_CURVE('',#2874,#2875,#1843,.T.);
#3630=EDGE_CURVE('',#2875,#2876,#280,.T.);
#3631=EDGE_CURVE('',#2815,#2876,#1844,.T.);
#3632=EDGE_CURVE('',#2860,#2850,#281,.T.);
#3633=EDGE_CURVE('',#2849,#2855,#282,.T.);
#3634=EDGE_CURVE('',#2877,#2847,#1845,.T.);
#3635=EDGE_CURVE('',#2877,#2861,#283,.T.);
#3636=EDGE_CURVE('',#2878,#2839,#1846,.T.);
#3637=EDGE_CURVE('',#2878,#2867,#284,.T.);
#3638=EDGE_CURVE('',#2879,#2835,#1847,.T.);
#3639=EDGE_CURVE('',#2879,#2880,#285,.T.);
#3640=EDGE_CURVE('',#2880,#2873,#286,.T.);
#3641=EDGE_CURVE('',#2834,#2881,#1848,.T.);
#3642=EDGE_CURVE('',#2882,#2881,#287,.T.);
#3643=EDGE_CURVE('',#2882,#2883,#288,.T.);
#3644=EDGE_CURVE('',#2884,#2883,#289,.T.);
#3645=EDGE_CURVE('',#2884,#2885,#1849,.T.);
#3646=EDGE_CURVE('',#2886,#2885,#290,.T.);
#3647=EDGE_CURVE('',#2886,#2887,#291,.T.);
#3648=EDGE_CURVE('',#2888,#2887,#292,.T.);
#3649=EDGE_CURVE('',#2888,#2817,#1850,.T.);
#3650=EDGE_CURVE('',#2876,#2889,#293,.T.);
#3651=EDGE_CURVE('',#2889,#2890,#294,.T.);
#3652=EDGE_CURVE('',#2820,#2890,#1851,.T.);
#3653=EDGE_CURVE('',#2872,#2891,#295,.T.);
#3654=EDGE_CURVE('',#2824,#2891,#1852,.T.);
#3655=EDGE_CURVE('',#2866,#2892,#296,.T.);
#3656=EDGE_CURVE('',#2828,#2892,#1853,.T.);
#3657=EDGE_CURVE('',#2893,#2894,#297,.T.);
#3658=EDGE_CURVE('',#2894,#2895,#298,.T.);
#3659=EDGE_CURVE('',#2895,#2896,#1854,.T.);
#3660=EDGE_CURVE('',#2896,#2897,#299,.T.);
#3661=EDGE_CURVE('',#2897,#2898,#300,.T.);
#3662=EDGE_CURVE('',#2893,#2898,#1855,.T.);
#3663=EDGE_CURVE('',#2899,#2899,#2496,.T.);
#3664=EDGE_CURVE('',#2899,#2844,#1856,.T.);
#3665=EDGE_CURVE('',#2900,#2900,#2497,.T.);
#3666=EDGE_CURVE('',#2900,#2843,#1857,.T.);
#3667=EDGE_CURVE('',#2893,#2901,#301,.T.);
#3668=EDGE_CURVE('',#2902,#2898,#302,.T.);
#3669=EDGE_CURVE('',#2903,#2902,#303,.T.);
#3670=EDGE_CURVE('',#2904,#2903,#1858,.T.);
#3671=EDGE_CURVE('',#2901,#2904,#304,.T.);
#3672=EDGE_CURVE('',#2859,#2851,#305,.T.);
#3673=EDGE_CURVE('',#2901,#2905,#306,.T.);
#3674=EDGE_CURVE('',#2905,#2894,#307,.T.);
#3675=EDGE_CURVE('',#2852,#2858,#308,.T.);
#3676=EDGE_CURVE('',#2906,#2904,#309,.T.);
#3677=EDGE_CURVE('',#2905,#2906,#2498,.F.);
#3678=EDGE_CURVE('',#2857,#2853,#310,.T.);
#3679=EDGE_CURVE('',#2903,#2907,#311,.T.);
#3680=EDGE_CURVE('',#2907,#2906,#1859,.T.);
#3681=EDGE_CURVE('',#2854,#2856,#312,.T.);
#3682=EDGE_CURVE('',#2897,#2908,#313,.T.);
#3683=EDGE_CURVE('',#2908,#2902,#314,.T.);
#3684=EDGE_CURVE('',#2909,#2892,#315,.T.);
#3685=EDGE_CURVE('',#2910,#2909,#316,.T.);
#3686=EDGE_CURVE('',#2911,#2910,#1860,.T.);
#3687=EDGE_CURVE('',#2912,#2911,#317,.T.);
#3688=EDGE_CURVE('',#2877,#2912,#318,.T.);
#3689=EDGE_CURVE('',#2865,#2909,#319,.T.);
#3690=EDGE_CURVE('',#2910,#2864,#320,.T.);
#3691=EDGE_CURVE('',#2863,#2911,#321,.T.);
#3692=EDGE_CURVE('',#2912,#2862,#322,.T.);
#3693=EDGE_CURVE('',#2913,#2891,#323,.T.);
#3694=EDGE_CURVE('',#2914,#2913,#324,.T.);
#3695=EDGE_CURVE('',#2915,#2914,#1861,.T.);
#3696=EDGE_CURVE('',#2916,#2915,#325,.T.);
#3697=EDGE_CURVE('',#2878,#2916,#326,.T.);
#3698=EDGE_CURVE('',#2871,#2913,#327,.T.);
#3699=EDGE_CURVE('',#2914,#2870,#328,.T.);
#3700=EDGE_CURVE('',#2869,#2915,#329,.T.);
#3701=EDGE_CURVE('',#2916,#2868,#330,.T.);
#3702=EDGE_CURVE('',#2917,#2890,#331,.T.);
#3703=EDGE_CURVE('',#2918,#2917,#332,.T.);
#3704=EDGE_CURVE('',#2919,#2918,#1862,.T.);
#3705=EDGE_CURVE('',#2920,#2919,#333,.T.);
#3706=EDGE_CURVE('',#2879,#2920,#334,.T.);
#3707=EDGE_CURVE('',#2889,#2921,#335,.T.);
#3708=EDGE_CURVE('',#2921,#2917,#336,.T.);
#3709=EDGE_CURVE('',#2922,#2921,#2499,.F.);
#3710=EDGE_CURVE('',#2918,#2922,#337,.T.);
#3711=EDGE_CURVE('',#2922,#2923,#1863,.T.);
#3712=EDGE_CURVE('',#2923,#2919,#338,.T.);
#3713=EDGE_CURVE('',#2920,#2924,#339,.T.);
#3714=EDGE_CURVE('',#2924,#2880,#340,.T.);
#3715=EDGE_CURVE('',#2924,#2923,#2500,.F.);
#3716=EDGE_CURVE('',#2923,#2874,#2501,.F.);
#3717=EDGE_CURVE('',#2874,#2924,#2502,.F.);
#3718=EDGE_CURVE('',#2907,#2908,#2503,.F.);
#3719=EDGE_CURVE('',#2908,#2925,#2504,.F.);
#3720=EDGE_CURVE('',#2925,#2907,#2505,.F.);
#3721=EDGE_CURVE('',#2921,#2875,#2506,.F.);
#3722=EDGE_CURVE('',#2875,#2922,#2507,.F.);
#3723=EDGE_CURVE('',#2926,#2905,#2508,.F.);
#3724=EDGE_CURVE('',#2906,#2926,#2509,.F.);
#3725=EDGE_CURVE('',#2926,#2925,#1864,.T.);
#3726=EDGE_CURVE('',#2895,#2926,#341,.T.);
#3727=EDGE_CURVE('',#2925,#2896,#342,.T.);
#3728=EDGE_CURVE('',#2927,#2928,#2510,.F.);
#3729=EDGE_CURVE('',#2929,#2927,#2511,.F.);
#3730=EDGE_CURVE('',#2928,#2929,#2512,.F.);
#3731=EDGE_CURVE('',#2930,#2931,#2513,.F.);
#3732=EDGE_CURVE('',#2932,#2930,#2514,.F.);
#3733=EDGE_CURVE('',#2931,#2932,#2515,.F.);
#3734=EDGE_CURVE('',#2933,#2934,#2516,.F.);
#3735=EDGE_CURVE('',#2935,#2933,#2517,.F.);
#3736=EDGE_CURVE('',#2934,#2935,#2518,.F.);
#3737=EDGE_CURVE('',#2928,#2935,#1865,.T.);
#3738=EDGE_CURVE('',#2933,#2927,#1866,.T.);
#3739=EDGE_CURVE('',#2887,#2934,#343,.T.);
#3740=EDGE_CURVE('',#2935,#2888,#344,.T.);
#3741=EDGE_CURVE('',#2936,#2937,#2519,.F.);
#3742=EDGE_CURVE('',#2938,#2936,#2520,.F.);
#3743=EDGE_CURVE('',#2937,#2938,#2521,.F.);
#3744=EDGE_CURVE('',#2936,#2932,#1867,.T.);
#3745=EDGE_CURVE('',#2930,#2938,#1868,.T.);
#3746=EDGE_CURVE('',#2934,#2937,#345,.T.);
#3747=EDGE_CURVE('',#2938,#2933,#346,.T.);
#3748=EDGE_CURVE('',#2885,#2936,#347,.T.);
#3749=EDGE_CURVE('',#2937,#2886,#348,.T.);
#3750=EDGE_CURVE('',#2883,#2931,#349,.T.);
#3751=EDGE_CURVE('',#2932,#2884,#350,.T.);
#3752=EDGE_CURVE('',#2931,#2929,#351,.T.);
#3753=EDGE_CURVE('',#2927,#2930,#352,.T.);
#3754=EDGE_CURVE('',#2881,#2928,#353,.T.);
#3755=EDGE_CURVE('',#2929,#2882,#354,.T.);
#4774=ORIENTED_EDGE('',*,*,#3504,.F.);
#4775=ORIENTED_EDGE('',*,*,#3505,.T.);
#4776=ORIENTED_EDGE('',*,*,#3506,.F.);
#4777=ORIENTED_EDGE('',*,*,#3505,.F.);
#4778=ORIENTED_EDGE('',*,*,#3507,.F.);
#4779=ORIENTED_EDGE('',*,*,#3508,.T.);
#4780=ORIENTED_EDGE('',*,*,#3509,.F.);
#4781=ORIENTED_EDGE('',*,*,#3508,.F.);
#4782=ORIENTED_EDGE('',*,*,#3510,.F.);
#4783=ORIENTED_EDGE('',*,*,#3511,.T.);
#4784=ORIENTED_EDGE('',*,*,#3512,.F.);
#4785=ORIENTED_EDGE('',*,*,#3511,.F.);
#4786=ORIENTED_EDGE('',*,*,#3513,.F.);
#4787=ORIENTED_EDGE('',*,*,#3514,.T.);
#4788=ORIENTED_EDGE('',*,*,#3515,.F.);
#4789=ORIENTED_EDGE('',*,*,#3514,.F.);
#4790=ORIENTED_EDGE('',*,*,#3516,.F.);
#4791=ORIENTED_EDGE('',*,*,#3517,.T.);
#4792=ORIENTED_EDGE('',*,*,#3518,.T.);
#4793=ORIENTED_EDGE('',*,*,#3519,.F.);
#4794=ORIENTED_EDGE('',*,*,#3520,.F.);
#4795=ORIENTED_EDGE('',*,*,#3521,.T.);
#4796=ORIENTED_EDGE('',*,*,#3522,.T.);
#4797=ORIENTED_EDGE('',*,*,#3517,.F.);
#4798=ORIENTED_EDGE('',*,*,#3523,.F.);
#4799=ORIENTED_EDGE('',*,*,#3524,.T.);
#4800=ORIENTED_EDGE('',*,*,#3525,.T.);
#4801=ORIENTED_EDGE('',*,*,#3521,.F.);
#4802=ORIENTED_EDGE('',*,*,#3526,.F.);
#4803=ORIENTED_EDGE('',*,*,#3527,.T.);
#4804=ORIENTED_EDGE('',*,*,#3528,.T.);
#4805=ORIENTED_EDGE('',*,*,#3524,.F.);
#4806=ORIENTED_EDGE('',*,*,#3529,.F.);
#4807=ORIENTED_EDGE('',*,*,#3530,.T.);
#4808=ORIENTED_EDGE('',*,*,#3531,.T.);
#4809=ORIENTED_EDGE('',*,*,#3527,.F.);
#4810=ORIENTED_EDGE('',*,*,#3532,.F.);
#4811=ORIENTED_EDGE('',*,*,#3519,.T.);
#4812=ORIENTED_EDGE('',*,*,#3533,.T.);
#4813=ORIENTED_EDGE('',*,*,#3530,.F.);
#4814=ORIENTED_EDGE('',*,*,#3533,.F.);
#4815=ORIENTED_EDGE('',*,*,#3518,.F.);
#4816=ORIENTED_EDGE('',*,*,#3522,.F.);
#4817=ORIENTED_EDGE('',*,*,#3525,.F.);
#4818=ORIENTED_EDGE('',*,*,#3528,.F.);
#4819=ORIENTED_EDGE('',*,*,#3531,.F.);
#4820=ORIENTED_EDGE('',*,*,#3534,.F.);
#4821=ORIENTED_EDGE('',*,*,#3535,.F.);
#4822=ORIENTED_EDGE('',*,*,#3536,.T.);
#4823=ORIENTED_EDGE('',*,*,#3537,.T.);
#4824=ORIENTED_EDGE('',*,*,#3538,.F.);
#4825=ORIENTED_EDGE('',*,*,#3539,.F.);
#4826=ORIENTED_EDGE('',*,*,#3540,.T.);
#4827=ORIENTED_EDGE('',*,*,#3541,.T.);
#4828=ORIENTED_EDGE('',*,*,#3536,.F.);
#4829=ORIENTED_EDGE('',*,*,#3542,.F.);
#4830=ORIENTED_EDGE('',*,*,#3543,.T.);
#4831=ORIENTED_EDGE('',*,*,#3544,.T.);
#4832=ORIENTED_EDGE('',*,*,#3540,.F.);
#4833=ORIENTED_EDGE('',*,*,#3545,.F.);
#4834=ORIENTED_EDGE('',*,*,#3546,.T.);
#4835=ORIENTED_EDGE('',*,*,#3547,.T.);
#4836=ORIENTED_EDGE('',*,*,#3543,.F.);
#4837=ORIENTED_EDGE('',*,*,#3548,.F.);
#4838=ORIENTED_EDGE('',*,*,#3549,.T.);
#4839=ORIENTED_EDGE('',*,*,#3550,.T.);
#4840=ORIENTED_EDGE('',*,*,#3546,.F.);
#4841=ORIENTED_EDGE('',*,*,#3551,.F.);
#4842=ORIENTED_EDGE('',*,*,#3538,.T.);
#4843=ORIENTED_EDGE('',*,*,#3552,.T.);
#4844=ORIENTED_EDGE('',*,*,#3549,.F.);
#4845=ORIENTED_EDGE('',*,*,#3552,.F.);
#4846=ORIENTED_EDGE('',*,*,#3537,.F.);
#4847=ORIENTED_EDGE('',*,*,#3541,.F.);
#4848=ORIENTED_EDGE('',*,*,#3544,.F.);
#4849=ORIENTED_EDGE('',*,*,#3547,.F.);
#4850=ORIENTED_EDGE('',*,*,#3550,.F.);
#4851=ORIENTED_EDGE('',*,*,#3553,.F.);
#4852=ORIENTED_EDGE('',*,*,#3553,.T.);
#4853=ORIENTED_EDGE('',*,*,#3554,.T.);
#4854=ORIENTED_EDGE('',*,*,#3555,.F.);
#4855=ORIENTED_EDGE('',*,*,#3554,.F.);
#4856=ORIENTED_EDGE('',*,*,#3534,.T.);
#4857=ORIENTED_EDGE('',*,*,#3556,.T.);
#4858=ORIENTED_EDGE('',*,*,#3557,.F.);
#4859=ORIENTED_EDGE('',*,*,#3556,.F.);
#4860=ORIENTED_EDGE('',*,*,#3558,.F.);
#4861=ORIENTED_EDGE('',*,*,#3559,.F.);
#4862=ORIENTED_EDGE('',*,*,#3560,.F.);
#4863=ORIENTED_EDGE('',*,*,#3561,.T.);
#4864=ORIENTED_EDGE('',*,*,#3562,.F.);
#4865=ORIENTED_EDGE('',*,*,#3563,.T.);
#4866=ORIENTED_EDGE('',*,*,#3564,.F.);
#4867=ORIENTED_EDGE('',*,*,#3565,.F.);
#4868=ORIENTED_EDGE('',*,*,#3566,.F.);
#4869=ORIENTED_EDGE('',*,*,#3567,.T.);
#4870=ORIENTED_EDGE('',*,*,#3568,.F.);
#4871=ORIENTED_EDGE('',*,*,#3569,.F.);
#4872=ORIENTED_EDGE('',*,*,#3570,.F.);
#4873=ORIENTED_EDGE('',*,*,#3571,.T.);
#4874=ORIENTED_EDGE('',*,*,#3572,.F.);
#4875=ORIENTED_EDGE('',*,*,#3573,.F.);
#4876=ORIENTED_EDGE('',*,*,#3574,.F.);
#4877=ORIENTED_EDGE('',*,*,#3575,.T.);
#4878=ORIENTED_EDGE('',*,*,#3576,.F.);
#4879=ORIENTED_EDGE('',*,*,#3577,.F.);
#4880=ORIENTED_EDGE('',*,*,#3578,.F.);
#4881=ORIENTED_EDGE('',*,*,#3579,.F.);
#4882=ORIENTED_EDGE('',*,*,#3580,.F.);
#4883=ORIENTED_EDGE('',*,*,#3581,.T.);
#4884=ORIENTED_EDGE('',*,*,#3582,.F.);
#4885=ORIENTED_EDGE('',*,*,#3583,.F.);
#4886=ORIENTED_EDGE('',*,*,#3584,.F.);
#4887=ORIENTED_EDGE('',*,*,#3585,.T.);
#4888=ORIENTED_EDGE('',*,*,#3586,.F.);
#4889=ORIENTED_EDGE('',*,*,#3555,.T.);
#4890=ORIENTED_EDGE('',*,*,#3587,.F.);
#4891=ORIENTED_EDGE('',*,*,#3557,.T.);
#4892=ORIENTED_EDGE('',*,*,#3588,.F.);
#4893=ORIENTED_EDGE('',*,*,#3561,.F.);
#4894=ORIENTED_EDGE('',*,*,#3589,.F.);
#4895=ORIENTED_EDGE('',*,*,#3575,.F.);
#4896=ORIENTED_EDGE('',*,*,#3590,.F.);
#4897=ORIENTED_EDGE('',*,*,#3581,.F.);
#4898=ORIENTED_EDGE('',*,*,#3591,.F.);
#4899=ORIENTED_EDGE('',*,*,#3563,.F.);
#4900=ORIENTED_EDGE('',*,*,#3592,.F.);
#4901=ORIENTED_EDGE('',*,*,#3585,.F.);
#4902=ORIENTED_EDGE('',*,*,#3593,.F.);
#4903=ORIENTED_EDGE('',*,*,#3567,.F.);
#4904=ORIENTED_EDGE('',*,*,#3594,.F.);
#4905=ORIENTED_EDGE('',*,*,#3595,.F.);
#4906=ORIENTED_EDGE('',*,*,#3596,.F.);
#4907=ORIENTED_EDGE('',*,*,#3571,.F.);
#4908=ORIENTED_EDGE('',*,*,#3597,.F.);
#4909=ORIENTED_EDGE('',*,*,#3598,.F.);
#4910=ORIENTED_EDGE('',*,*,#3599,.F.);
#4911=ORIENTED_EDGE('',*,*,#3595,.T.);
#4912=ORIENTED_EDGE('',*,*,#3600,.T.);
#4913=ORIENTED_EDGE('',*,*,#3601,.F.);
#4914=ORIENTED_EDGE('',*,*,#3602,.F.);
#4915=ORIENTED_EDGE('',*,*,#3603,.F.);
#4916=ORIENTED_EDGE('',*,*,#3604,.F.);
#4917=ORIENTED_EDGE('',*,*,#3605,.F.);
#4918=ORIENTED_EDGE('',*,*,#3572,.T.);
#4919=ORIENTED_EDGE('',*,*,#3596,.T.);
#4920=ORIENTED_EDGE('',*,*,#3599,.T.);
#4921=ORIENTED_EDGE('',*,*,#3606,.T.);
#4922=ORIENTED_EDGE('',*,*,#3607,.F.);
#4923=ORIENTED_EDGE('',*,*,#3608,.F.);
#4924=ORIENTED_EDGE('',*,*,#3609,.F.);
#4925=ORIENTED_EDGE('',*,*,#3610,.F.);
#4926=ORIENTED_EDGE('',*,*,#3611,.F.);
#4927=ORIENTED_EDGE('',*,*,#3612,.T.);
#4928=ORIENTED_EDGE('',*,*,#3568,.T.);
#4929=ORIENTED_EDGE('',*,*,#3593,.T.);
#4930=ORIENTED_EDGE('',*,*,#3584,.T.);
#4931=ORIENTED_EDGE('',*,*,#3613,.T.);
#4932=ORIENTED_EDGE('',*,*,#3614,.F.);
#4933=ORIENTED_EDGE('',*,*,#3615,.F.);
#4934=ORIENTED_EDGE('',*,*,#3616,.F.);
#4935=ORIENTED_EDGE('',*,*,#3617,.F.);
#4936=ORIENTED_EDGE('',*,*,#3618,.F.);
#4937=ORIENTED_EDGE('',*,*,#3619,.T.);
#4938=ORIENTED_EDGE('',*,*,#3564,.T.);
#4939=ORIENTED_EDGE('',*,*,#3591,.T.);
#4940=ORIENTED_EDGE('',*,*,#3580,.T.);
#4941=ORIENTED_EDGE('',*,*,#3620,.T.);
#4942=ORIENTED_EDGE('',*,*,#3621,.F.);
#4943=ORIENTED_EDGE('',*,*,#3622,.F.);
#4944=ORIENTED_EDGE('',*,*,#3623,.F.);
#4945=ORIENTED_EDGE('',*,*,#3624,.F.);
#4946=ORIENTED_EDGE('',*,*,#3625,.F.);
#4947=ORIENTED_EDGE('',*,*,#3626,.T.);
#4948=ORIENTED_EDGE('',*,*,#3558,.T.);
#4949=ORIENTED_EDGE('',*,*,#3588,.T.);
#4950=ORIENTED_EDGE('',*,*,#3574,.T.);
#4951=ORIENTED_EDGE('',*,*,#3627,.F.);
#4952=ORIENTED_EDGE('',*,*,#3628,.T.);
#4953=ORIENTED_EDGE('',*,*,#3629,.T.);
#4954=ORIENTED_EDGE('',*,*,#3630,.T.);
#4955=ORIENTED_EDGE('',*,*,#3631,.F.);
#4956=ORIENTED_EDGE('',*,*,#3573,.T.);
#4957=ORIENTED_EDGE('',*,*,#3612,.F.);
#4958=ORIENTED_EDGE('',*,*,#3632,.T.);
#4959=ORIENTED_EDGE('',*,*,#3600,.F.);
#4960=ORIENTED_EDGE('',*,*,#3633,.T.);
#4961=ORIENTED_EDGE('',*,*,#3606,.F.);
#4962=ORIENTED_EDGE('',*,*,#3598,.T.);
#4963=ORIENTED_EDGE('',*,*,#3634,.F.);
#4964=ORIENTED_EDGE('',*,*,#3635,.T.);
#4965=ORIENTED_EDGE('',*,*,#3613,.F.);
#4966=ORIENTED_EDGE('',*,*,#3583,.T.);
#4967=ORIENTED_EDGE('',*,*,#3636,.F.);
#4968=ORIENTED_EDGE('',*,*,#3637,.T.);
#4969=ORIENTED_EDGE('',*,*,#3620,.F.);
#4970=ORIENTED_EDGE('',*,*,#3579,.T.);
#4971=ORIENTED_EDGE('',*,*,#3638,.F.);
#4972=ORIENTED_EDGE('',*,*,#3639,.T.);
#4973=ORIENTED_EDGE('',*,*,#3640,.T.);
#4974=ORIENTED_EDGE('',*,*,#3627,.T.);
#4975=ORIENTED_EDGE('',*,*,#3577,.T.);
#4976=ORIENTED_EDGE('',*,*,#3641,.T.);
#4977=ORIENTED_EDGE('',*,*,#3642,.F.);
#4978=ORIENTED_EDGE('',*,*,#3643,.T.);
#4979=ORIENTED_EDGE('',*,*,#3644,.F.);
#4980=ORIENTED_EDGE('',*,*,#3645,.T.);
#4981=ORIENTED_EDGE('',*,*,#3646,.F.);
#4982=ORIENTED_EDGE('',*,*,#3647,.T.);
#4983=ORIENTED_EDGE('',*,*,#3648,.F.);
#4984=ORIENTED_EDGE('',*,*,#3649,.T.);
#4985=ORIENTED_EDGE('',*,*,#3559,.T.);
#4986=ORIENTED_EDGE('',*,*,#3631,.T.);
#4987=ORIENTED_EDGE('',*,*,#3650,.T.);
#4988=ORIENTED_EDGE('',*,*,#3651,.T.);
#4989=ORIENTED_EDGE('',*,*,#3652,.F.);
#4990=ORIENTED_EDGE('',*,*,#3565,.T.);
#4991=ORIENTED_EDGE('',*,*,#3626,.F.);
#4992=ORIENTED_EDGE('',*,*,#3653,.T.);
#4993=ORIENTED_EDGE('',*,*,#3654,.F.);
#4994=ORIENTED_EDGE('',*,*,#3569,.T.);
#4995=ORIENTED_EDGE('',*,*,#3619,.F.);
#4996=ORIENTED_EDGE('',*,*,#3655,.T.);
#4997=ORIENTED_EDGE('',*,*,#3656,.F.);
#4998=ORIENTED_EDGE('',*,*,#3657,.T.);
#4999=ORIENTED_EDGE('',*,*,#3658,.T.);
#5000=ORIENTED_EDGE('',*,*,#3659,.T.);
#5001=ORIENTED_EDGE('',*,*,#3660,.T.);
#5002=ORIENTED_EDGE('',*,*,#3661,.T.);
#5003=ORIENTED_EDGE('',*,*,#3662,.F.);
#5004=ORIENTED_EDGE('',*,*,#3663,.F.);
#5005=ORIENTED_EDGE('',*,*,#3664,.T.);
#5006=ORIENTED_EDGE('',*,*,#3587,.T.);
#5007=ORIENTED_EDGE('',*,*,#3664,.F.);
#5008=ORIENTED_EDGE('',*,*,#3665,.F.);
#5009=ORIENTED_EDGE('',*,*,#3666,.T.);
#5010=ORIENTED_EDGE('',*,*,#3586,.T.);
#5011=ORIENTED_EDGE('',*,*,#3666,.F.);
#5012=ORIENTED_EDGE('',*,*,#3667,.F.);
#5013=ORIENTED_EDGE('',*,*,#3662,.T.);
#5014=ORIENTED_EDGE('',*,*,#3668,.F.);
#5015=ORIENTED_EDGE('',*,*,#3669,.F.);
#5016=ORIENTED_EDGE('',*,*,#3670,.F.);
#5017=ORIENTED_EDGE('',*,*,#3671,.F.);
#5018=ORIENTED_EDGE('',*,*,#3601,.T.);
#5019=ORIENTED_EDGE('',*,*,#3632,.F.);
#5020=ORIENTED_EDGE('',*,*,#3611,.T.);
#5021=ORIENTED_EDGE('',*,*,#3672,.T.);
#5022=ORIENTED_EDGE('',*,*,#3667,.T.);
#5023=ORIENTED_EDGE('',*,*,#3673,.T.);
#5024=ORIENTED_EDGE('',*,*,#3674,.T.);
#5025=ORIENTED_EDGE('',*,*,#3657,.F.);
#5026=ORIENTED_EDGE('',*,*,#3602,.T.);
#5027=ORIENTED_EDGE('',*,*,#3672,.F.);
#5028=ORIENTED_EDGE('',*,*,#3610,.T.);
#5029=ORIENTED_EDGE('',*,*,#3675,.F.);
#5030=ORIENTED_EDGE('',*,*,#3671,.T.);
#5031=ORIENTED_EDGE('',*,*,#3676,.F.);
#5032=ORIENTED_EDGE('',*,*,#3677,.F.);
#5033=ORIENTED_EDGE('',*,*,#3673,.F.);
#5034=ORIENTED_EDGE('',*,*,#3603,.T.);
#5035=ORIENTED_EDGE('',*,*,#3675,.T.);
#5036=ORIENTED_EDGE('',*,*,#3609,.T.);
#5037=ORIENTED_EDGE('',*,*,#3678,.T.);
#5038=ORIENTED_EDGE('',*,*,#3506,.T.);
#5039=ORIENTED_EDGE('',*,*,#3515,.T.);
#5040=ORIENTED_EDGE('',*,*,#3663,.T.);
#5041=ORIENTED_EDGE('',*,*,#3670,.T.);
#5042=ORIENTED_EDGE('',*,*,#3679,.T.);
#5043=ORIENTED_EDGE('',*,*,#3680,.T.);
#5044=ORIENTED_EDGE('',*,*,#3676,.T.);
#5045=ORIENTED_EDGE('',*,*,#3604,.T.);
#5046=ORIENTED_EDGE('',*,*,#3678,.F.);
#5047=ORIENTED_EDGE('',*,*,#3608,.T.);
#5048=ORIENTED_EDGE('',*,*,#3681,.F.);
#5049=ORIENTED_EDGE('',*,*,#3605,.T.);
#5050=ORIENTED_EDGE('',*,*,#3681,.T.);
#5051=ORIENTED_EDGE('',*,*,#3607,.T.);
#5052=ORIENTED_EDGE('',*,*,#3633,.F.);
#5053=ORIENTED_EDGE('',*,*,#3668,.T.);
#5054=ORIENTED_EDGE('',*,*,#3661,.F.);
#5055=ORIENTED_EDGE('',*,*,#3682,.T.);
#5056=ORIENTED_EDGE('',*,*,#3683,.T.);
#5057=ORIENTED_EDGE('',*,*,#3570,.T.);
#5058=ORIENTED_EDGE('',*,*,#3656,.T.);
#5059=ORIENTED_EDGE('',*,*,#3684,.F.);
#5060=ORIENTED_EDGE('',*,*,#3685,.F.);
#5061=ORIENTED_EDGE('',*,*,#3686,.F.);
#5062=ORIENTED_EDGE('',*,*,#3687,.F.);
#5063=ORIENTED_EDGE('',*,*,#3688,.F.);
#5064=ORIENTED_EDGE('',*,*,#3634,.T.);
#5065=ORIENTED_EDGE('',*,*,#3597,.T.);
#5066=ORIENTED_EDGE('',*,*,#3594,.T.);
#5067=ORIENTED_EDGE('',*,*,#3684,.T.);
#5068=ORIENTED_EDGE('',*,*,#3655,.F.);
#5069=ORIENTED_EDGE('',*,*,#3618,.T.);
#5070=ORIENTED_EDGE('',*,*,#3689,.T.);
#5071=ORIENTED_EDGE('',*,*,#3685,.T.);
#5072=ORIENTED_EDGE('',*,*,#3689,.F.);
#5073=ORIENTED_EDGE('',*,*,#3617,.T.);
#5074=ORIENTED_EDGE('',*,*,#3690,.F.);
#5075=ORIENTED_EDGE('',*,*,#3686,.T.);
#5076=ORIENTED_EDGE('',*,*,#3690,.T.);
#5077=ORIENTED_EDGE('',*,*,#3616,.T.);
#5078=ORIENTED_EDGE('',*,*,#3691,.T.);
#5079=ORIENTED_EDGE('',*,*,#3687,.T.);
#5080=ORIENTED_EDGE('',*,*,#3691,.F.);
#5081=ORIENTED_EDGE('',*,*,#3615,.T.);
#5082=ORIENTED_EDGE('',*,*,#3692,.F.);
#5083=ORIENTED_EDGE('',*,*,#3688,.T.);
#5084=ORIENTED_EDGE('',*,*,#3692,.T.);
#5085=ORIENTED_EDGE('',*,*,#3614,.T.);
#5086=ORIENTED_EDGE('',*,*,#3635,.F.);
#5087=ORIENTED_EDGE('',*,*,#3566,.T.);
#5088=ORIENTED_EDGE('',*,*,#3654,.T.);
#5089=ORIENTED_EDGE('',*,*,#3693,.F.);
#5090=ORIENTED_EDGE('',*,*,#3694,.F.);
#5091=ORIENTED_EDGE('',*,*,#3695,.F.);
#5092=ORIENTED_EDGE('',*,*,#3696,.F.);
#5093=ORIENTED_EDGE('',*,*,#3697,.F.);
#5094=ORIENTED_EDGE('',*,*,#3636,.T.);
#5095=ORIENTED_EDGE('',*,*,#3582,.T.);
#5096=ORIENTED_EDGE('',*,*,#3592,.T.);
#5097=ORIENTED_EDGE('',*,*,#3693,.T.);
#5098=ORIENTED_EDGE('',*,*,#3653,.F.);
#5099=ORIENTED_EDGE('',*,*,#3625,.T.);
#5100=ORIENTED_EDGE('',*,*,#3698,.T.);
#5101=ORIENTED_EDGE('',*,*,#3694,.T.);
#5102=ORIENTED_EDGE('',*,*,#3698,.F.);
#5103=ORIENTED_EDGE('',*,*,#3624,.T.);
#5104=ORIENTED_EDGE('',*,*,#3699,.F.);
#5105=ORIENTED_EDGE('',*,*,#3695,.T.);
#5106=ORIENTED_EDGE('',*,*,#3699,.T.);
#5107=ORIENTED_EDGE('',*,*,#3623,.T.);
#5108=ORIENTED_EDGE('',*,*,#3700,.T.);
#5109=ORIENTED_EDGE('',*,*,#3509,.T.);
#5110=ORIENTED_EDGE('',*,*,#3512,.T.);
#5111=ORIENTED_EDGE('',*,*,#3665,.T.);
#5112=ORIENTED_EDGE('',*,*,#3696,.T.);
#5113=ORIENTED_EDGE('',*,*,#3700,.F.);
#5114=ORIENTED_EDGE('',*,*,#3622,.T.);
#5115=ORIENTED_EDGE('',*,*,#3701,.F.);
#5116=ORIENTED_EDGE('',*,*,#3697,.T.);
#5117=ORIENTED_EDGE('',*,*,#3701,.T.);
#5118=ORIENTED_EDGE('',*,*,#3621,.T.);
#5119=ORIENTED_EDGE('',*,*,#3637,.F.);
#5120=ORIENTED_EDGE('',*,*,#3562,.T.);
#5121=ORIENTED_EDGE('',*,*,#3652,.T.);
#5122=ORIENTED_EDGE('',*,*,#3702,.F.);
#5123=ORIENTED_EDGE('',*,*,#3703,.F.);
#5124=ORIENTED_EDGE('',*,*,#3704,.F.);
#5125=ORIENTED_EDGE('',*,*,#3705,.F.);
#5126=ORIENTED_EDGE('',*,*,#3706,.F.);
#5127=ORIENTED_EDGE('',*,*,#3638,.T.);
#5128=ORIENTED_EDGE('',*,*,#3578,.T.);
#5129=ORIENTED_EDGE('',*,*,#3590,.T.);
#5130=ORIENTED_EDGE('',*,*,#3702,.T.);
#5131=ORIENTED_EDGE('',*,*,#3651,.F.);
#5132=ORIENTED_EDGE('',*,*,#3707,.T.);
#5133=ORIENTED_EDGE('',*,*,#3708,.T.);
#5134=ORIENTED_EDGE('',*,*,#3703,.T.);
#5135=ORIENTED_EDGE('',*,*,#3708,.F.);
#5136=ORIENTED_EDGE('',*,*,#3709,.F.);
#5137=ORIENTED_EDGE('',*,*,#3710,.F.);
#5138=ORIENTED_EDGE('',*,*,#3704,.T.);
#5139=ORIENTED_EDGE('',*,*,#3710,.T.);
#5140=ORIENTED_EDGE('',*,*,#3711,.T.);
#5141=ORIENTED_EDGE('',*,*,#3712,.T.);
#5142=ORIENTED_EDGE('',*,*,#3706,.T.);
#5143=ORIENTED_EDGE('',*,*,#3713,.T.);
#5144=ORIENTED_EDGE('',*,*,#3714,.T.);
#5145=ORIENTED_EDGE('',*,*,#3639,.F.);
#5146=ORIENTED_EDGE('',*,*,#3705,.T.);
#5147=ORIENTED_EDGE('',*,*,#3712,.F.);
#5148=ORIENTED_EDGE('',*,*,#3715,.F.);
#5149=ORIENTED_EDGE('',*,*,#3713,.F.);
#5150=ORIENTED_EDGE('',*,*,#3716,.T.);
#5151=ORIENTED_EDGE('',*,*,#3717,.T.);
#5152=ORIENTED_EDGE('',*,*,#3715,.T.);
#5153=ORIENTED_EDGE('',*,*,#3718,.T.);
#5154=ORIENTED_EDGE('',*,*,#3719,.T.);
#5155=ORIENTED_EDGE('',*,*,#3720,.T.);
#5156=ORIENTED_EDGE('',*,*,#3709,.T.);
#5157=ORIENTED_EDGE('',*,*,#3721,.T.);
#5158=ORIENTED_EDGE('',*,*,#3722,.T.);
#5159=ORIENTED_EDGE('',*,*,#3716,.F.);
#5160=ORIENTED_EDGE('',*,*,#3711,.F.);
#5161=ORIENTED_EDGE('',*,*,#3722,.F.);
#5162=ORIENTED_EDGE('',*,*,#3629,.F.);
#5163=ORIENTED_EDGE('',*,*,#3650,.F.);
#5164=ORIENTED_EDGE('',*,*,#3630,.F.);
#5165=ORIENTED_EDGE('',*,*,#3721,.F.);
#5166=ORIENTED_EDGE('',*,*,#3707,.F.);
#5167=ORIENTED_EDGE('',*,*,#3723,.T.);
#5168=ORIENTED_EDGE('',*,*,#3677,.T.);
#5169=ORIENTED_EDGE('',*,*,#3724,.T.);
#5170=ORIENTED_EDGE('',*,*,#3724,.F.);
#5171=ORIENTED_EDGE('',*,*,#3680,.F.);
#5172=ORIENTED_EDGE('',*,*,#3720,.F.);
#5173=ORIENTED_EDGE('',*,*,#3725,.F.);
#5174=ORIENTED_EDGE('',*,*,#3658,.F.);
#5175=ORIENTED_EDGE('',*,*,#3674,.F.);
#5176=ORIENTED_EDGE('',*,*,#3723,.F.);
#5177=ORIENTED_EDGE('',*,*,#3726,.F.);
#5178=ORIENTED_EDGE('',*,*,#3660,.F.);
#5179=ORIENTED_EDGE('',*,*,#3727,.F.);
#5180=ORIENTED_EDGE('',*,*,#3719,.F.);
#5181=ORIENTED_EDGE('',*,*,#3682,.F.);
#5182=ORIENTED_EDGE('',*,*,#3669,.T.);
#5183=ORIENTED_EDGE('',*,*,#3683,.F.);
#5184=ORIENTED_EDGE('',*,*,#3718,.F.);
#5185=ORIENTED_EDGE('',*,*,#3679,.F.);
#5186=ORIENTED_EDGE('',*,*,#3640,.F.);
#5187=ORIENTED_EDGE('',*,*,#3714,.F.);
#5188=ORIENTED_EDGE('',*,*,#3717,.F.);
#5189=ORIENTED_EDGE('',*,*,#3628,.F.);
#5190=ORIENTED_EDGE('',*,*,#3726,.T.);
#5191=ORIENTED_EDGE('',*,*,#3725,.T.);
#5192=ORIENTED_EDGE('',*,*,#3727,.T.);
#5193=ORIENTED_EDGE('',*,*,#3659,.F.);
#5194=ORIENTED_EDGE('',*,*,#3728,.F.);
#5195=ORIENTED_EDGE('',*,*,#3729,.F.);
#5196=ORIENTED_EDGE('',*,*,#3730,.F.);
#5197=ORIENTED_EDGE('',*,*,#3731,.F.);
#5198=ORIENTED_EDGE('',*,*,#3732,.F.);
#5199=ORIENTED_EDGE('',*,*,#3733,.F.);
#5200=ORIENTED_EDGE('',*,*,#3734,.F.);
#5201=ORIENTED_EDGE('',*,*,#3735,.F.);
#5202=ORIENTED_EDGE('',*,*,#3736,.F.);
#5203=ORIENTED_EDGE('',*,*,#3728,.T.);
#5204=ORIENTED_EDGE('',*,*,#3737,.T.);
#5205=ORIENTED_EDGE('',*,*,#3735,.T.);
#5206=ORIENTED_EDGE('',*,*,#3738,.T.);
#5207=ORIENTED_EDGE('',*,*,#3648,.T.);
#5208=ORIENTED_EDGE('',*,*,#3739,.T.);
#5209=ORIENTED_EDGE('',*,*,#3736,.T.);
#5210=ORIENTED_EDGE('',*,*,#3740,.T.);
#5211=ORIENTED_EDGE('',*,*,#3741,.F.);
#5212=ORIENTED_EDGE('',*,*,#3742,.F.);
#5213=ORIENTED_EDGE('',*,*,#3743,.F.);
#5214=ORIENTED_EDGE('',*,*,#3742,.T.);
#5215=ORIENTED_EDGE('',*,*,#3744,.T.);
#5216=ORIENTED_EDGE('',*,*,#3732,.T.);
#5217=ORIENTED_EDGE('',*,*,#3745,.T.);
#5218=ORIENTED_EDGE('',*,*,#3734,.T.);
#5219=ORIENTED_EDGE('',*,*,#3746,.T.);
#5220=ORIENTED_EDGE('',*,*,#3743,.T.);
#5221=ORIENTED_EDGE('',*,*,#3747,.T.);
#5222=ORIENTED_EDGE('',*,*,#3646,.T.);
#5223=ORIENTED_EDGE('',*,*,#3748,.T.);
#5224=ORIENTED_EDGE('',*,*,#3741,.T.);
#5225=ORIENTED_EDGE('',*,*,#3749,.T.);
#5226=ORIENTED_EDGE('',*,*,#3644,.T.);
#5227=ORIENTED_EDGE('',*,*,#3750,.T.);
#5228=ORIENTED_EDGE('',*,*,#3733,.T.);
#5229=ORIENTED_EDGE('',*,*,#3751,.T.);
#5230=ORIENTED_EDGE('',*,*,#3731,.T.);
#5231=ORIENTED_EDGE('',*,*,#3752,.T.);
#5232=ORIENTED_EDGE('',*,*,#3729,.T.);
#5233=ORIENTED_EDGE('',*,*,#3753,.T.);
#5234=ORIENTED_EDGE('',*,*,#3642,.T.);
#5235=ORIENTED_EDGE('',*,*,#3754,.T.);
#5236=ORIENTED_EDGE('',*,*,#3730,.T.);
#5237=ORIENTED_EDGE('',*,*,#3755,.T.);
#5238=ORIENTED_EDGE('',*,*,#3749,.F.);
#5239=ORIENTED_EDGE('',*,*,#3746,.F.);
#5240=ORIENTED_EDGE('',*,*,#3739,.F.);
#5241=ORIENTED_EDGE('',*,*,#3647,.F.);
#5242=ORIENTED_EDGE('',*,*,#3560,.T.);
#5243=ORIENTED_EDGE('',*,*,#3649,.F.);
#5244=ORIENTED_EDGE('',*,*,#3740,.F.);
#5245=ORIENTED_EDGE('',*,*,#3737,.F.);
#5246=ORIENTED_EDGE('',*,*,#3754,.F.);
#5247=ORIENTED_EDGE('',*,*,#3641,.F.);
#5248=ORIENTED_EDGE('',*,*,#3576,.T.);
#5249=ORIENTED_EDGE('',*,*,#3589,.T.);
#5250=ORIENTED_EDGE('',*,*,#3745,.F.);
#5251=ORIENTED_EDGE('',*,*,#3753,.F.);
#5252=ORIENTED_EDGE('',*,*,#3738,.F.);
#5253=ORIENTED_EDGE('',*,*,#3747,.F.);
#5254=ORIENTED_EDGE('',*,*,#3535,.T.);
#5255=ORIENTED_EDGE('',*,*,#3551,.T.);
#5256=ORIENTED_EDGE('',*,*,#3548,.T.);
#5257=ORIENTED_EDGE('',*,*,#3545,.T.);
#5258=ORIENTED_EDGE('',*,*,#3542,.T.);
#5259=ORIENTED_EDGE('',*,*,#3539,.T.);
#5260=ORIENTED_EDGE('',*,*,#3516,.T.);
#5261=ORIENTED_EDGE('',*,*,#3532,.T.);
#5262=ORIENTED_EDGE('',*,*,#3529,.T.);
#5263=ORIENTED_EDGE('',*,*,#3526,.T.);
#5264=ORIENTED_EDGE('',*,*,#3523,.T.);
#5265=ORIENTED_EDGE('',*,*,#3520,.T.);
#5266=ORIENTED_EDGE('',*,*,#3513,.T.);
#5267=ORIENTED_EDGE('',*,*,#3510,.T.);
#5268=ORIENTED_EDGE('',*,*,#3507,.T.);
#5269=ORIENTED_EDGE('',*,*,#3504,.T.);
#5270=ORIENTED_EDGE('',*,*,#3750,.F.);
#5271=ORIENTED_EDGE('',*,*,#3643,.F.);
#5272=ORIENTED_EDGE('',*,*,#3755,.F.);
#5273=ORIENTED_EDGE('',*,*,#3752,.F.);
#5274=ORIENTED_EDGE('',*,*,#3748,.F.);
#5275=ORIENTED_EDGE('',*,*,#3645,.F.);
#5276=ORIENTED_EDGE('',*,*,#3751,.F.);
#5277=ORIENTED_EDGE('',*,*,#3744,.F.);
#6012=CYLINDRICAL_SURFACE('',#6789,0.15);
#6013=CYLINDRICAL_SURFACE('',#6792,0.15);
#6014=CYLINDRICAL_SURFACE('',#6795,0.15);
#6015=CYLINDRICAL_SURFACE('',#6798,0.15);
#6016=CYLINDRICAL_SURFACE('',#6817,0.17);
#6017=CYLINDRICAL_SURFACE('',#6819,0.17);
#6018=CYLINDRICAL_SURFACE('',#6843,0.4);
#6019=CYLINDRICAL_SURFACE('',#6845,0.4);
#6020=CYLINDRICAL_SURFACE('',#6869,0.1);
#6021=CYLINDRICAL_SURFACE('',#6873,0.1);
#6022=CYLINDRICAL_SURFACE('',#6887,0.3);
#6023=CYLINDRICAL_SURFACE('',#6892,0.3);
#6249=ADVANCED_FACE('',(#918),#6012,.F.);
#6250=ADVANCED_FACE('',(#919),#6013,.F.);
#6251=ADVANCED_FACE('',(#920),#6014,.F.);
#6252=ADVANCED_FACE('',(#921),#6015,.F.);
#6253=ADVANCED_FACE('',(#922),#703,.F.);
#6254=ADVANCED_FACE('',(#923),#704,.F.);
#6255=ADVANCED_FACE('',(#924),#705,.F.);
#6256=ADVANCED_FACE('',(#925),#706,.F.);
#6257=ADVANCED_FACE('',(#926),#707,.F.);
#6258=ADVANCED_FACE('',(#927),#708,.F.);
#6259=ADVANCED_FACE('',(#928,#603),#709,.F.);
#6260=ADVANCED_FACE('',(#929),#710,.F.);
#6261=ADVANCED_FACE('',(#930),#711,.F.);
#6262=ADVANCED_FACE('',(#931),#712,.F.);
#6263=ADVANCED_FACE('',(#932),#713,.F.);
#6264=ADVANCED_FACE('',(#933),#714,.F.);
#6265=ADVANCED_FACE('',(#934),#715,.F.);
#6266=ADVANCED_FACE('',(#935,#604),#716,.F.);
#6267=ADVANCED_FACE('',(#936),#6016,.F.);
#6268=ADVANCED_FACE('',(#937),#6017,.F.);
#6269=ADVANCED_FACE('',(#938),#717,.F.);
#6270=ADVANCED_FACE('',(#939),#718,.F.);
#6271=ADVANCED_FACE('',(#940),#719,.F.);
#6272=ADVANCED_FACE('',(#941),#720,.F.);
#6273=ADVANCED_FACE('',(#942),#721,.F.);
#6274=ADVANCED_FACE('',(#943),#722,.F.);
#6275=ADVANCED_FACE('',(#944),#723,.F.);
#6276=ADVANCED_FACE('',(#945,#605),#724,.F.);
#6277=ADVANCED_FACE('',(#946,#606),#725,.F.);
#6278=ADVANCED_FACE('',(#947),#726,.F.);
#6279=ADVANCED_FACE('',(#948),#727,.F.);
#6280=ADVANCED_FACE('',(#949),#728,.F.);
#6281=ADVANCED_FACE('',(#950),#729,.F.);
#6282=ADVANCED_FACE('',(#951),#730,.F.);
#6283=ADVANCED_FACE('',(#952),#731,.T.);
#6284=ADVANCED_FACE('',(#953),#732,.T.);
#6285=ADVANCED_FACE('',(#954),#733,.T.);
#6286=ADVANCED_FACE('',(#955),#734,.T.);
#6287=ADVANCED_FACE('',(#956),#735,.T.);
#6288=ADVANCED_FACE('',(#957,#607),#736,.F.);
#6289=ADVANCED_FACE('',(#958),#6018,.T.);
#6290=ADVANCED_FACE('',(#959),#6019,.T.);
#6291=ADVANCED_FACE('',(#960),#737,.T.);
#6292=ADVANCED_FACE('',(#961),#123,.T.);
#6293=ADVANCED_FACE('',(#962),#124,.T.);
#6294=ADVANCED_FACE('',(#963),#125,.T.);
#6295=ADVANCED_FACE('',(#964),#126,.T.);
#6296=ADVANCED_FACE('',(#965,#608,#609,#610),#738,.F.);
#6297=ADVANCED_FACE('',(#966),#739,.F.);
#6298=ADVANCED_FACE('',(#967),#127,.T.);
#6299=ADVANCED_FACE('',(#968),#128,.T.);
#6300=ADVANCED_FACE('',(#969),#129,.T.);
#6301=ADVANCED_FACE('',(#970),#740,.T.);
#6302=ADVANCED_FACE('',(#971),#130,.T.);
#6303=ADVANCED_FACE('',(#972),#131,.T.);
#6304=ADVANCED_FACE('',(#973),#741,.F.);
#6305=ADVANCED_FACE('',(#974),#132,.T.);
#6306=ADVANCED_FACE('',(#975),#133,.T.);
#6307=ADVANCED_FACE('',(#976),#742,.T.);
#6308=ADVANCED_FACE('',(#977),#134,.T.);
#6309=ADVANCED_FACE('',(#978),#135,.T.);
#6310=ADVANCED_FACE('',(#979,#611,#612,#613),#743,.F.);
#6311=ADVANCED_FACE('',(#980),#136,.T.);
#6312=ADVANCED_FACE('',(#981),#137,.T.);
#6313=ADVANCED_FACE('',(#982),#744,.T.);
#6314=ADVANCED_FACE('',(#983),#138,.T.);
#6315=ADVANCED_FACE('',(#984),#139,.T.);
#6316=ADVANCED_FACE('',(#985),#745,.F.);
#6317=ADVANCED_FACE('',(#986),#140,.T.);
#6318=ADVANCED_FACE('',(#987),#141,.T.);
#6319=ADVANCED_FACE('',(#988),#83,.F.);
#6320=ADVANCED_FACE('',(#989),#84,.F.);
#6321=ADVANCED_FACE('',(#990),#85,.F.);
#6322=ADVANCED_FACE('',(#991),#6020,.F.);
#6323=ADVANCED_FACE('',(#992),#142,.T.);
#6324=ADVANCED_FACE('',(#993),#86,.F.);
#6325=ADVANCED_FACE('',(#994),#6021,.F.);
#6326=ADVANCED_FACE('',(#995),#143,.T.);
#6327=ADVANCED_FACE('',(#996),#144,.T.);
#6328=ADVANCED_FACE('',(#997),#145,.T.);
#6329=ADVANCED_FACE('',(#998),#146,.T.);
#6330=ADVANCED_FACE('',(#999),#746,.T.);
#6331=ADVANCED_FACE('',(#1000),#87,.T.);
#6332=ADVANCED_FACE('',(#1001),#88,.T.);
#6333=ADVANCED_FACE('',(#1002),#89,.T.);
#6334=ADVANCED_FACE('',(#1003),#6022,.T.);
#6335=ADVANCED_FACE('',(#1004),#147,.F.);
#6336=ADVANCED_FACE('',(#1005),#90,.T.);
#6337=ADVANCED_FACE('',(#1006),#6023,.T.);
#6338=ADVANCED_FACE('',(#1007),#148,.F.);
#6339=ADVANCED_FACE('',(#1008),#149,.F.);
#6340=ADVANCED_FACE('',(#1009),#150,.F.);
#6341=ADVANCED_FACE('',(#1010),#151,.F.);
#6342=ADVANCED_FACE('',(#1011),#152,.F.);
#6343=ADVANCED_FACE('',(#1012),#153,.F.);
#6344=ADVANCED_FACE('',(#1013),#747,.F.);
#6345=ADVANCED_FACE('',(#1014,#614,#615,#616,#617,#618,#619),#748,.T.);
#6346=ADVANCED_FACE('',(#1015),#154,.F.);
#6347=ADVANCED_FACE('',(#1016),#749,.F.);
#6490=CLOSED_SHELL('',(#6249,#6250,#6251,#6252,#6253,#6254,#6255,#6256,
#6257,#6258,#6259,#6260,#6261,#6262,#6263,#6264,#6265,#6266,#6267,#6268,
#6269,#6270,#6271,#6272,#6273,#6274,#6275,#6276,#6277,#6278,#6279,#6280,
#6281,#6282,#6283,#6284,#6285,#6286,#6287,#6288,#6289,#6290,#6291,#6292,
#6293,#6294,#6295,#6296,#6297,#6298,#6299,#6300,#6301,#6302,#6303,#6304,
#6305,#6306,#6307,#6308,#6309,#6310,#6311,#6312,#6313,#6314,#6315,#6316,
#6317,#6318,#6319,#6320,#6321,#6322,#6323,#6324,#6325,#6326,#6327,#6328,
#6329,#6330,#6331,#6332,#6333,#6334,#6335,#6336,#6337,#6338,#6339,#6340,
#6341,#6342,#6343,#6344,#6345,#6346,#6347));
#6788=AXIS2_PLACEMENT_3D('',#10631,#7626,#7627);
#6789=AXIS2_PLACEMENT_3D('',#10632,#7628,#7629);
#6790=AXIS2_PLACEMENT_3D('',#10634,#7630,#7631);
#6791=AXIS2_PLACEMENT_3D('',#10637,#7633,#7634);
#6792=AXIS2_PLACEMENT_3D('',#10638,#7635,#7636);
#6793=AXIS2_PLACEMENT_3D('',#10640,#7637,#7638);
#6794=AXIS2_PLACEMENT_3D('',#10643,#7640,#7641);
#6795=AXIS2_PLACEMENT_3D('',#10644,#7642,#7643);
#6796=AXIS2_PLACEMENT_3D('',#10646,#7644,#7645);
#6797=AXIS2_PLACEMENT_3D('',#10649,#7647,#7648);
#6798=AXIS2_PLACEMENT_3D('',#10650,#7649,#7650);
#6799=AXIS2_PLACEMENT_3D('',#10652,#7651,#7652);
#6800=AXIS2_PLACEMENT_3D('',#10655,#7654,#7655);
#6801=AXIS2_PLACEMENT_3D('',#10656,#7656,#7657);
#6802=AXIS2_PLACEMENT_3D('',#10665,#7662,#7663);
#6803=AXIS2_PLACEMENT_3D('',#10671,#7667,#7668);
#6804=AXIS2_PLACEMENT_3D('',#10677,#7672,#7673);
#6805=AXIS2_PLACEMENT_3D('',#10683,#7677,#7678);
#6806=AXIS2_PLACEMENT_3D('',#10689,#7682,#7683);
#6807=AXIS2_PLACEMENT_3D('',#10692,#7686,#7687);
#6808=AXIS2_PLACEMENT_3D('',#10694,#7688,#7689);
#6809=AXIS2_PLACEMENT_3D('',#10695,#7690,#7691);
#6810=AXIS2_PLACEMENT_3D('',#10704,#7696,#7697);
#6811=AXIS2_PLACEMENT_3D('',#10710,#7701,#7702);
#6812=AXIS2_PLACEMENT_3D('',#10716,#7706,#7707);
#6813=AXIS2_PLACEMENT_3D('',#10722,#7711,#7712);
#6814=AXIS2_PLACEMENT_3D('',#10728,#7716,#7717);
#6815=AXIS2_PLACEMENT_3D('',#10731,#7720,#7721);
#6816=AXIS2_PLACEMENT_3D('',#10733,#7722,#7723);
#6817=AXIS2_PLACEMENT_3D('',#10734,#7724,#7725);
#6818=AXIS2_PLACEMENT_3D('',#10737,#7727,#7728);
#6819=AXIS2_PLACEMENT_3D('',#10738,#7729,#7730);
#6820=AXIS2_PLACEMENT_3D('',#10741,#7732,#7733);
#6821=AXIS2_PLACEMENT_3D('',#10742,#7734,#7735);
#6822=AXIS2_PLACEMENT_3D('',#10751,#7740,#7741);
#6823=AXIS2_PLACEMENT_3D('',#10760,#7746,#7747);
#6824=AXIS2_PLACEMENT_3D('',#10769,#7752,#7753);
#6825=AXIS2_PLACEMENT_3D('',#10778,#7758,#7759);
#6826=AXIS2_PLACEMENT_3D('',#10787,#7764,#7765);
#6827=AXIS2_PLACEMENT_3D('',#10796,#7770,#7771);
#6828=AXIS2_PLACEMENT_3D('',#10805,#7776,#7777);
#6829=AXIS2_PLACEMENT_3D('',#10807,#7778,#7779);
#6830=AXIS2_PLACEMENT_3D('',#10808,#7780,#7781);
#6831=AXIS2_PLACEMENT_3D('',#10810,#7782,#7783);
#6832=AXIS2_PLACEMENT_3D('',#10811,#7784,#7785);
#6833=AXIS2_PLACEMENT_3D('',#10814,#7788,#7789);
#6834=AXIS2_PLACEMENT_3D('',#10817,#7792,#7793);
#6835=AXIS2_PLACEMENT_3D('',#10820,#7796,#7797);
#6836=AXIS2_PLACEMENT_3D('',#10826,#7801,#7802);
#6837=AXIS2_PLACEMENT_3D('',#10832,#7806,#7807);
#6838=AXIS2_PLACEMENT_3D('',#10909,#7810,#7811);
#6839=AXIS2_PLACEMENT_3D('',#10987,#7815,#7816);
#6840=AXIS2_PLACEMENT_3D('',#11065,#7820,#7821);
#6841=AXIS2_PLACEMENT_3D('',#11143,#7825,#7826);
#6842=AXIS2_PLACEMENT_3D('',#11159,#7830,#7831);
#6843=AXIS2_PLACEMENT_3D('',#11483,#7843,#7844);
#6844=AXIS2_PLACEMENT_3D('',#11485,#7845,#7846);
#6845=AXIS2_PLACEMENT_3D('',#11487,#7848,#7849);
#6846=AXIS2_PLACEMENT_3D('',#11489,#7850,#7851);
#6847=AXIS2_PLACEMENT_3D('',#11491,#7853,#7854);
#6848=AXIS2_PLACEMENT_3D('',#11659,#7856,#7857);
#6849=AXIS2_PLACEMENT_3D('',#11660,#7858,#7859);
#6850=AXIS2_PLACEMENT_3D('',#11665,#7860,#7861);
#6851=AXIS2_PLACEMENT_3D('',#11737,#7863,#7864);
#6852=AXIS2_PLACEMENT_3D('',#11855,#7866,#7867);
#6853=AXIS2_PLACEMENT_3D('',#11900,#7868,#7869);
#6854=AXIS2_PLACEMENT_3D('',#12018,#7871,#7872);
#6855=AXIS2_PLACEMENT_3D('',#12063,#7873,#7874);
#6856=AXIS2_PLACEMENT_3D('',#12183,#7876,#7877);
#6857=AXIS2_PLACEMENT_3D('',#12188,#7878,#7879);
#6858=AXIS2_PLACEMENT_3D('',#12240,#7881,#7882);
#6859=AXIS2_PLACEMENT_3D('',#12241,#7883,#7884);
#6860=AXIS2_PLACEMENT_3D('',#12242,#7885,#7886);
#6861=AXIS2_PLACEMENT_3D('',#12243,#7887,#7888);
#6862=AXIS2_PLACEMENT_3D('',#12244,#7889,#7890);
#6863=AXIS2_PLACEMENT_3D('',#12245,#7891,#7892);
#6864=AXIS2_PLACEMENT_3D('',#12247,#7893,#7894);
#6865=AXIS2_PLACEMENT_3D('',#12248,#7895,#7896);
#6866=AXIS2_PLACEMENT_3D('',#12249,#7897,#7898);
#6867=AXIS2_PLACEMENT_3D('',#12250,#7899,#7900);
#6868=AXIS2_PLACEMENT_3D('',#12251,#7901,#7902);
#6869=AXIS2_PLACEMENT_3D('',#12252,#7903,#7904);
#6870=AXIS2_PLACEMENT_3D('',#12273,#7905,#7906);
#6871=AXIS2_PLACEMENT_3D('',#12275,#7907,#7908);
#6872=AXIS2_PLACEMENT_3D('',#12276,#7909,#7910);
#6873=AXIS2_PLACEMENT_3D('',#12277,#7911,#7912);
#6874=AXIS2_PLACEMENT_3D('',#12367,#7914,#7915);
#6875=AXIS2_PLACEMENT_3D('',#12368,#7916,#7917);
#6876=AXIS2_PLACEMENT_3D('',#12371,#7918,#7919);
#6877=AXIS2_PLACEMENT_3D('',#12373,#7920,#7921);
#6878=AXIS2_PLACEMENT_3D('',#12374,#7922,#7923);
#6879=AXIS2_PLACEMENT_3D('',#12375,#7924,#7925);
#6880=AXIS2_PLACEMENT_3D('',#12378,#7926,#7927);
#6881=AXIS2_PLACEMENT_3D('',#12380,#7928,#7929);
#6882=AXIS2_PLACEMENT_3D('',#12381,#7930,#7931);
#6883=AXIS2_PLACEMENT_3D('',#12382,#7932,#7933);
#6884=AXIS2_PLACEMENT_3D('',#12385,#7934,#7935);
#6885=AXIS2_PLACEMENT_3D('',#12387,#7936,#7937);
#6886=AXIS2_PLACEMENT_3D('',#12388,#7938,#7939);
#6887=AXIS2_PLACEMENT_3D('',#12389,#7940,#7941);
#6888=AXIS2_PLACEMENT_3D('',#12420,#7944,#7945);
#6889=AXIS2_PLACEMENT_3D('',#12423,#7946,#7947);
#6890=AXIS2_PLACEMENT_3D('',#12425,#7948,#7949);
#6891=AXIS2_PLACEMENT_3D('',#12426,#7950,#7951);
#6892=AXIS2_PLACEMENT_3D('',#12427,#7952,#7953);
#6893=AXIS2_PLACEMENT_3D('',#12607,#7956,#7957);
#6894=AXIS2_PLACEMENT_3D('',#12608,#7958,#7959);
#6895=AXIS2_PLACEMENT_3D('',#12625,#7960,#7961);
#7626=DIRECTION('axis',(0.,0.,1.));
#7627=DIRECTION('refdir',(1.,0.,0.));
#7628=DIRECTION('center_axis',(0.,0.,-1.));
#7629=DIRECTION('ref_axis',(1.,0.,0.));
#7630=DIRECTION('center_axis',(1.01338750660366E-31,-1.26069923670246E-19,
-1.));
#7631=DIRECTION('ref_axis',(1.,0.,0.));
#7632=DIRECTION('',(0.,0.,-1.));
#7633=DIRECTION('center_axis',(-1.01338750660366E-31,1.26069923670246E-19,
1.));
#7634=DIRECTION('ref_axis',(1.,0.,0.));
#7635=DIRECTION('center_axis',(0.,0.,-1.));
#7636=DIRECTION('ref_axis',(1.,0.,0.));
#7637=DIRECTION('center_axis',(1.01338750660366E-31,-1.26069923670246E-19,
-1.));
#7638=DIRECTION('ref_axis',(1.,0.,0.));
#7639=DIRECTION('',(0.,0.,-1.));
#7640=DIRECTION('center_axis',(-1.01338750660366E-31,1.26069923670246E-19,
1.));
#7641=DIRECTION('ref_axis',(1.,0.,0.));
#7642=DIRECTION('center_axis',(0.,0.,-1.));
#7643=DIRECTION('ref_axis',(1.,0.,0.));
#7644=DIRECTION('center_axis',(1.01338750660366E-31,-1.26069923670246E-19,
-1.));
#7645=DIRECTION('ref_axis',(1.,0.,0.));
#7646=DIRECTION('',(0.,0.,-1.));
#7647=DIRECTION('center_axis',(-1.01338750660366E-31,1.26069923670246E-19,
1.));
#7648=DIRECTION('ref_axis',(1.,0.,0.));
#7649=DIRECTION('center_axis',(0.,0.,-1.));
#7650=DIRECTION('ref_axis',(1.,0.,0.));
#7651=DIRECTION('center_axis',(1.01338750660366E-31,-1.26069923670246E-19,
-1.));
#7652=DIRECTION('ref_axis',(1.,0.,0.));
#7653=DIRECTION('',(0.,0.,-1.));
#7654=DIRECTION('center_axis',(-1.01338750660366E-31,1.26069923670246E-19,
1.));
#7655=DIRECTION('ref_axis',(1.,0.,0.));
#7656=DIRECTION('center_axis',(0.86602540378444,0.499999999999998,0.));
#7657=DIRECTION('ref_axis',(0.499999999999998,-0.86602540378444,0.));
#7658=DIRECTION('',(0.499999999999998,-0.86602540378444,1.09179756551649E-19));
#7659=DIRECTION('',(0.,0.,-1.));
#7660=DIRECTION('',(0.499999999999998,-0.86602540378444,0.));
#7661=DIRECTION('',(0.,0.,-1.));
#7662=DIRECTION('center_axis',(1.60246890531963E-16,1.,0.));
#7663=DIRECTION('ref_axis',(1.,-1.60246890531963E-16,0.));
#7664=DIRECTION('',(1.,-1.60246890531963E-16,1.01358952973624E-31));
#7665=DIRECTION('',(0.,0.,-1.));
#7666=DIRECTION('',(1.,-1.60246890531963E-16,0.));
#7667=DIRECTION('center_axis',(-0.86602540378444,0.499999999999998,0.));
#7668=DIRECTION('ref_axis',(0.499999999999998,0.86602540378444,0.));
#7669=DIRECTION('',(0.499999999999998,0.86602540378444,-1.09179756551548E-19));
#7670=DIRECTION('',(0.,0.,-1.));
#7671=DIRECTION('',(0.499999999999998,0.86602540378444,0.));
#7672=DIRECTION('center_axis',(-0.86602540378444,-0.499999999999998,0.));
#7673=DIRECTION('ref_axis',(-0.499999999999998,0.86602540378444,0.));
#7674=DIRECTION('',(-0.499999999999998,0.86602540378444,-1.09179756551649E-19));
#7675=DIRECTION('',(0.,0.,-1.));
#7676=DIRECTION('',(-0.499999999999998,0.86602540378444,0.));
#7677=DIRECTION('center_axis',(-1.60246890531963E-16,-1.,0.));
#7678=DIRECTION('ref_axis',(-1.,1.60246890531963E-16,0.));
#7679=DIRECTION('',(-1.,1.60246890531963E-16,-1.01358952973624E-31));
#7680=DIRECTION('',(0.,0.,-1.));
#7681=DIRECTION('',(-1.,1.60246890531963E-16,0.));
#7682=DIRECTION('center_axis',(0.86602540378444,-0.499999999999998,0.));
#7683=DIRECTION('ref_axis',(-0.499999999999998,-0.86602540378444,0.));
#7684=DIRECTION('',(-0.499999999999998,-0.86602540378444,1.09179756551548E-19));
#7685=DIRECTION('',(-0.499999999999998,-0.86602540378444,0.));
#7686=DIRECTION('center_axis',(0.,0.,-1.));
#7687=DIRECTION('ref_axis',(-1.,0.,0.));
#7688=DIRECTION('center_axis',(0.,0.,1.));
#7689=DIRECTION('ref_axis',(1.,0.,0.));
#7690=DIRECTION('center_axis',(0.866025403784439,0.5,0.));
#7691=DIRECTION('ref_axis',(0.5,-0.866025403784439,0.));
#7692=DIRECTION('',(0.5,-0.866025403784439,1.09179756551649E-19));
#7693=DIRECTION('',(0.,0.,-1.));
#7694=DIRECTION('',(0.5,-0.866025403784439,0.));
#7695=DIRECTION('',(0.,0.,-1.));
#7696=DIRECTION('center_axis',(1.60246890531964E-16,1.,0.));
#7697=DIRECTION('ref_axis',(1.,-1.60246890531964E-16,0.));
#7698=DIRECTION('',(1.,-1.60246890531964E-16,1.01358952973624E-31));
#7699=DIRECTION('',(0.,0.,-1.));
#7700=DIRECTION('',(1.,-1.60246890531964E-16,0.));
#7701=DIRECTION('center_axis',(-0.866025403784438,0.5,0.));
#7702=DIRECTION('ref_axis',(0.5,0.866025403784438,0.));
#7703=DIRECTION('',(0.5,0.866025403784438,-1.09179756551547E-19));
#7704=DIRECTION('',(0.,0.,-1.));
#7705=DIRECTION('',(0.5,0.866025403784438,0.));
#7706=DIRECTION('center_axis',(-0.866025403784439,-0.499999999999999,0.));
#7707=DIRECTION('ref_axis',(-0.499999999999999,0.866025403784439,0.));
#7708=DIRECTION('',(-0.499999999999999,0.866025403784439,-1.09179756551649E-19));
#7709=DIRECTION('',(0.,0.,-1.));
#7710=DIRECTION('',(-0.499999999999999,0.866025403784439,0.));
#7711=DIRECTION('center_axis',(-1.60246890531964E-16,-1.,0.));
#7712=DIRECTION('ref_axis',(-1.,1.60246890531964E-16,0.));
#7713=DIRECTION('',(-1.,1.60246890531964E-16,-1.01358952973624E-31));
#7714=DIRECTION('',(0.,0.,-1.));
#7715=DIRECTION('',(-1.,1.60246890531964E-16,0.));
#7716=DIRECTION('center_axis',(0.866025403784439,-0.5,0.));
#7717=DIRECTION('ref_axis',(-0.5,-0.866025403784439,0.));
#7718=DIRECTION('',(-0.5,-0.866025403784439,1.09179756551547E-19));
#7719=DIRECTION('',(-0.5,-0.866025403784439,0.));
#7720=DIRECTION('center_axis',(0.,0.,-1.));
#7721=DIRECTION('ref_axis',(-1.,0.,0.));
#7722=DIRECTION('center_axis',(0.,0.,1.));
#7723=DIRECTION('ref_axis',(1.,0.,0.));
#7724=DIRECTION('center_axis',(0.,0.,-1.));
#7725=DIRECTION('ref_axis',(1.,0.,0.));
#7726=DIRECTION('',(0.,0.,-1.));
#7727=DIRECTION('center_axis',(0.,0.,1.));
#7728=DIRECTION('ref_axis',(1.,0.,0.));
#7729=DIRECTION('center_axis',(0.,0.,-1.));
#7730=DIRECTION('ref_axis',(1.,0.,0.));
#7731=DIRECTION('',(0.,0.,-1.));
#7732=DIRECTION('center_axis',(0.,0.,1.));
#7733=DIRECTION('ref_axis',(1.,0.,0.));
#7734=DIRECTION('center_axis',(0.,-1.,0.));
#7735=DIRECTION('ref_axis',(-1.,0.,0.));
#7736=DIRECTION('',(0.0523359562429438,0.,0.998629534754574));
#7737=DIRECTION('',(1.,0.,0.));
#7738=DIRECTION('',(-0.0523359562429438,0.,-0.998629534754574));
#7739=DIRECTION('',(1.,0.,0.));
#7740=DIRECTION('center_axis',(0.,-1.,0.));
#7741=DIRECTION('ref_axis',(-1.,0.,0.));
#7742=DIRECTION('',(0.,0.,-1.));
#7743=DIRECTION('',(1.,0.,0.));
#7744=DIRECTION('',(0.,0.,1.));
#7745=DIRECTION('',(1.,0.,0.));
#7746=DIRECTION('center_axis',(0.,-1.,0.));
#7747=DIRECTION('ref_axis',(-1.,0.,0.));
#7748=DIRECTION('',(0.,0.,-1.));
#7749=DIRECTION('',(1.,0.,0.));
#7750=DIRECTION('',(0.,0.,1.));
#7751=DIRECTION('',(1.,0.,0.));
#7752=DIRECTION('center_axis',(0.,-1.,0.));
#7753=DIRECTION('ref_axis',(-1.,0.,0.));
#7754=DIRECTION('',(0.,0.,-1.));
#7755=DIRECTION('',(1.,0.,0.));
#7756=DIRECTION('',(0.,0.,1.));
#7757=DIRECTION('',(1.,0.,0.));
#7758=DIRECTION('center_axis',(0.,1.,0.));
#7759=DIRECTION('ref_axis',(1.,0.,0.));
#7760=DIRECTION('',(-0.0523359562429438,0.,-0.998629534754574));
#7761=DIRECTION('',(-1.,0.,0.));
#7762=DIRECTION('',(0.0523359562429438,0.,0.998629534754574));
#7763=DIRECTION('',(-1.,0.,0.));
#7764=DIRECTION('center_axis',(0.,1.,0.));
#7765=DIRECTION('ref_axis',(1.,0.,0.));
#7766=DIRECTION('',(0.,0.,1.));
#7767=DIRECTION('',(-1.,0.,0.));
#7768=DIRECTION('',(0.,0.,-1.));
#7769=DIRECTION('',(-1.,0.,0.));
#7770=DIRECTION('center_axis',(0.,1.,0.));
#7771=DIRECTION('ref_axis',(1.,0.,0.));
#7772=DIRECTION('',(0.,0.,1.));
#7773=DIRECTION('',(-1.,0.,0.));
#7774=DIRECTION('',(0.,0.,-1.));
#7775=DIRECTION('',(-1.,0.,0.));
#7776=DIRECTION('center_axis',(0.,0.,1.));
#7777=DIRECTION('ref_axis',(1.,0.,0.));
#7778=DIRECTION('center_axis',(0.,0.,1.));
#7779=DIRECTION('ref_axis',(1.,0.,0.));
#7780=DIRECTION('center_axis',(0.,0.,1.));
#7781=DIRECTION('ref_axis',(1.,0.,0.));
#7782=DIRECTION('center_axis',(0.,0.,1.));
#7783=DIRECTION('ref_axis',(1.,0.,0.));
#7784=DIRECTION('center_axis',(0.,0.,1.));
#7785=DIRECTION('ref_axis',(1.,0.,0.));
#7786=DIRECTION('',(0.,1.,0.));
#7787=DIRECTION('',(0.,-1.,0.));
#7788=DIRECTION('center_axis',(0.,0.,1.));
#7789=DIRECTION('ref_axis',(1.,0.,0.));
#7790=DIRECTION('',(0.,-1.,0.));
#7791=DIRECTION('',(0.,1.,0.));
#7792=DIRECTION('center_axis',(0.,0.,1.));
#7793=DIRECTION('ref_axis',(1.,0.,0.));
#7794=DIRECTION('',(0.,-1.,0.));
#7795=DIRECTION('',(0.,1.,0.));
#7796=DIRECTION('center_axis',(0.,0.,1.));
#7797=DIRECTION('ref_axis',(1.,0.,0.));
#7798=DIRECTION('',(0.,-1.,0.));
#7799=DIRECTION('',(-1.,0.,0.));
#7800=DIRECTION('',(0.,1.,0.));
#7801=DIRECTION('center_axis',(0.,1.,0.));
#7802=DIRECTION('ref_axis',(1.,0.,0.));
#7803=DIRECTION('',(0.,0.,1.));
#7804=DIRECTION('',(-1.,0.,0.));
#7805=DIRECTION('',(0.,0.,-1.));
#7806=DIRECTION('center_axis',(-1.,0.,0.));
#7807=DIRECTION('ref_axis',(0.,-1.,0.));
#7808=DIRECTION('',(0.,-1.,0.));
#7809=DIRECTION('',(0.,-1.,1.26069923670246E-19));
#7810=DIRECTION('center_axis',(1.,0.,0.));
#7811=DIRECTION('ref_axis',(0.,1.,0.));
#7812=DIRECTION('',(0.,1.,0.));
#7813=DIRECTION('',(0.,1.,-1.26069923670246E-19));
#7814=DIRECTION('',(0.,1.,0.));
#7815=DIRECTION('center_axis',(1.,0.,0.));
#7816=DIRECTION('ref_axis',(0.,1.,0.));
#7817=DIRECTION('',(0.,1.,0.));
#7818=DIRECTION('',(0.,1.,-1.26069923670246E-19));
#7819=DIRECTION('',(0.,1.,0.));
#7820=DIRECTION('center_axis',(1.,0.,0.));
#7821=DIRECTION('ref_axis',(0.,1.,0.));
#7822=DIRECTION('',(0.,1.,0.));
#7823=DIRECTION('',(0.,1.,-1.26069923670246E-19));
#7824=DIRECTION('',(0.,1.,0.));
#7825=DIRECTION('center_axis',(0.998629534754574,0.,-0.0523359562429438));
#7826=DIRECTION('ref_axis',(-0.0523359562429438,0.,-0.998629534754574));
#7827=DIRECTION('',(0.,-1.,0.));
#7828=DIRECTION('',(6.6070447339401E-21,-1.,1.26069923670246E-19));
#7829=DIRECTION('',(0.,-1.,0.));
#7830=DIRECTION('center_axis',(0.,0.,1.));
#7831=DIRECTION('ref_axis',(1.,0.,0.));
#7832=DIRECTION('',(0.,-1.,0.));
#7833=DIRECTION('',(0.,-1.,0.));
#7834=DIRECTION('',(0.,-1.,0.));
#7835=DIRECTION('',(0.,1.,0.));
#7836=DIRECTION('',(0.,-1.,0.));
#7837=DIRECTION('',(0.,1.,0.));
#7838=DIRECTION('',(0.,-1.,0.));
#7839=DIRECTION('',(0.,-1.,0.));
#7840=DIRECTION('',(0.,-1.,0.));
#7841=DIRECTION('',(0.,1.,0.));
#7842=DIRECTION('',(0.,1.,0.));
#7843=DIRECTION('center_axis',(0.,0.,1.));
#7844=DIRECTION('ref_axis',(1.,0.,0.));
#7845=DIRECTION('center_axis',(-1.01338750660366E-31,1.26069923670246E-19,
1.));
#7846=DIRECTION('ref_axis',(1.,0.,0.));
#7847=DIRECTION('',(0.,0.,-1.));
#7848=DIRECTION('center_axis',(0.,0.,1.));
#7849=DIRECTION('ref_axis',(1.,0.,0.));
#7850=DIRECTION('center_axis',(-1.01338750660366E-31,1.26069923670246E-19,
1.));
#7851=DIRECTION('ref_axis',(1.,0.,0.));
#7852=DIRECTION('',(0.,0.,-1.));
#7853=DIRECTION('center_axis',(1.,0.,0.));
#7854=DIRECTION('ref_axis',(0.,1.,0.));
#7855=DIRECTION('',(0.,1.,-1.26069923670246E-19));
#7856=DIRECTION('center_axis',(0.995216631131787,0.0976926666577189,1.18580395612125E-14));
#7857=DIRECTION('ref_axis',(0.0975341006448478,-0.993601284365854,0.0569524970297685));
#7858=DIRECTION('center_axis',(-1.01338750660366E-31,1.26069923670246E-19,
1.));
#7859=DIRECTION('ref_axis',(1.,0.,1.01338750660366E-31));
#7860=DIRECTION('center_axis',(-1.01338750660366E-31,1.26069923670246E-19,
1.));
#7861=DIRECTION('ref_axis',(1.,0.,1.01338750660366E-31));
#7862=DIRECTION('',(-6.60704473394009E-21,-1.,1.26069923670246E-19));
#7863=DIRECTION('center_axis',(-1.,0.,0.));
#7864=DIRECTION('ref_axis',(0.,-1.,0.));
#7865=DIRECTION('',(0.,-1.,1.26069923670246E-19));
#7866=DIRECTION('center_axis',(-1.01338750660366E-31,1.26069923670246E-19,
1.));
#7867=DIRECTION('ref_axis',(1.,0.,1.01338750660366E-31));
#7868=DIRECTION('center_axis',(-1.,0.,0.));
#7869=DIRECTION('ref_axis',(0.,-1.,0.));
#7870=DIRECTION('',(0.,-1.,1.26069923670246E-19));
#7871=DIRECTION('center_axis',(-1.01338750660366E-31,1.26069923670246E-19,
1.));
#7872=DIRECTION('ref_axis',(1.,0.,1.01338750660366E-31));
#7873=DIRECTION('center_axis',(-1.,0.,0.));
#7874=DIRECTION('ref_axis',(0.,-1.,0.));
#7875=DIRECTION('',(0.,-1.,1.26069923670246E-19));
#7876=DIRECTION('center_axis',(-0.982258063247475,0.187534256031586,1.45403402392141E-15));
#7877=DIRECTION('ref_axis',(1.48029736616688E-15,0.,1.));
#7878=DIRECTION('center_axis',(-1.01338750660366E-31,1.26069923670246E-19,
1.));
#7879=DIRECTION('ref_axis',(1.,0.,1.01338750660366E-31));
#7880=DIRECTION('',(-6.6070447339401E-21,1.,-1.26069923670246E-19));
#7881=DIRECTION('center_axis',(-0.982258063247479,-0.187534256031562,9.14061384143289E-15));
#7882=DIRECTION('ref_axis',(-0.187187393251729,0.980441281772238,0.0607928680392112));
#7883=DIRECTION('center_axis',(-0.45173408531537,0.373496730537872,-0.810207694632559));
#7884=DIRECTION('ref_axis',(-0.624418441188311,0.516273298501642,0.586142893463867));
#7885=DIRECTION('center_axis',(-2.96465769266614E-15,1.,0.));
#7886=DIRECTION('ref_axis',(0.,0.,1.));
#7887=DIRECTION('center_axis',(0.0522655346583812,-0.0518587053130894,0.997285810873755));
#7888=DIRECTION('ref_axis',(-0.998629534754574,0.,0.0523359562429445));
#7889=DIRECTION('center_axis',(0.377681861983732,-0.843372107574977,0.38220400219391));
#7890=DIRECTION('ref_axis',(0.592794689304902,0.537329962094562,0.599892463836113));
#7891=DIRECTION('center_axis',(0.995216631131786,-0.0976926666577302,0.));
#7892=DIRECTION('ref_axis',(0.,0.,1.));
#7893=DIRECTION('center_axis',(-0.0522650609395843,-0.052032719242908,0.997276771780618));
#7894=DIRECTION('ref_axis',(0.0975341006448596,0.993601284365853,0.0569524970297681));
#7895=DIRECTION('center_axis',(1.55158195278682E-16,1.,-2.96059473233375E-15));
#7896=DIRECTION('ref_axis',(0.998629534754574,0.,0.0523359562429438));
#7897=DIRECTION('center_axis',(-0.45173408531537,-0.373496730537869,-0.810207694632561));
#7898=DIRECTION('ref_axis',(-0.624418441188315,-0.516273298501641,0.586142893463864));
#7899=DIRECTION('center_axis',(0.0522655346583823,0.0518587053130918,0.997285810873755));
#7900=DIRECTION('ref_axis',(-0.187187393251729,-0.980441281772238,0.0607928680392122));
#7901=DIRECTION('center_axis',(-2.71526841737693E-16,-1.,-5.18104078158406E-15));
#7902=DIRECTION('ref_axis',(-0.998629534754574,0.,0.0523359562429439));
#7903=DIRECTION('center_axis',(-6.6070447339401E-21,1.,-1.26069923670246E-19));
#7904=DIRECTION('ref_axis',(-0.688354575693753,0.,0.725374371012289));
#7905=DIRECTION('center_axis',(-0.377681861983722,-0.843372107574983,-0.382204002193908));
#7906=DIRECTION('ref_axis',(0.592794689304909,-0.537329962094554,0.599892463836112));
#7907=DIRECTION('center_axis',(-0.0522650609395818,0.0520327192429072,0.997276771780618));
#7908=DIRECTION('ref_axis',(0.998629534754574,0.,0.0523359562429431));
#7909=DIRECTION('center_axis',(2.96465769266612E-15,-1.,0.));
#7910=DIRECTION('ref_axis',(0.,0.,1.));
#7911=DIRECTION('center_axis',(-6.60704473394009E-21,-1.,1.26069923670246E-19));
#7912=DIRECTION('ref_axis',(0.688354575693758,0.,0.725374371012284));
#7913=DIRECTION('',(6.60704473394009E-21,1.,-1.26069923670246E-19));
#7914=DIRECTION('center_axis',(-0.998629534754574,0.,-0.0523359562429438));
#7915=DIRECTION('ref_axis',(-0.0523359562429438,0.,0.998629534754574));
#7916=DIRECTION('center_axis',(-0.45173408531537,0.373496730537872,-0.81020769463256));
#7917=DIRECTION('ref_axis',(-0.624418441188311,0.516273298501643,0.586142893463866));
#7918=DIRECTION('center_axis',(-2.96465769266614E-15,1.,0.));
#7919=DIRECTION('ref_axis',(0.,0.,1.));
#7920=DIRECTION('center_axis',(-0.982258063247479,-0.187534256031562,9.14061384143289E-15));
#7921=DIRECTION('ref_axis',(-0.187187393251729,0.980441281772238,0.0607928680392111));
#7922=DIRECTION('center_axis',(0.0522655346583812,-0.0518587053130894,0.997285810873755));
#7923=DIRECTION('ref_axis',(-0.998629534754574,0.,0.0523359562429445));
#7924=DIRECTION('center_axis',(0.377681861983731,-0.843372107574978,0.38220400219391));
#7925=DIRECTION('ref_axis',(0.592794689304906,0.537329962094559,0.599892463836111));
#7926=DIRECTION('center_axis',(0.995216631131786,-0.0976926666577302,0.));
#7927=DIRECTION('ref_axis',(0.,0.,1.));
#7928=DIRECTION('center_axis',(1.55158195278682E-16,1.,-2.96059473233375E-15));
#7929=DIRECTION('ref_axis',(0.998629534754574,0.,0.0523359562429438));
#7930=DIRECTION('center_axis',(-0.0522650609395843,-0.052032719242908,0.997276771780618));
#7931=DIRECTION('ref_axis',(0.0975341006448596,0.993601284365853,0.0569524970297681));
#7932=DIRECTION('center_axis',(-0.45173408531537,-0.373496730537868,-0.810207694632561));
#7933=DIRECTION('ref_axis',(-0.624418441188315,-0.516273298501641,0.586142893463864));
#7934=DIRECTION('center_axis',(-0.982258063247475,0.187534256031586,1.45403402392141E-15));
#7935=DIRECTION('ref_axis',(1.48029736616688E-15,0.,1.));
#7936=DIRECTION('center_axis',(-2.71526841737693E-16,-1.,-5.18104078158406E-15));
#7937=DIRECTION('ref_axis',(-0.998629534754574,0.,0.0523359562429439));
#7938=DIRECTION('center_axis',(0.0522655346583823,0.0518587053130918,0.997285810873755));
#7939=DIRECTION('ref_axis',(-0.187187393251729,-0.980441281772238,0.0607928680392122));
#7940=DIRECTION('center_axis',(-6.6070447339401E-21,1.,-1.26069923670246E-19));
#7941=DIRECTION('ref_axis',(-0.688354575693753,0.,0.725374371012289));
#7942=DIRECTION('',(6.6070447339401E-21,-1.,1.26069923670246E-19));
#7943=DIRECTION('',(-6.6070447339401E-21,1.,-1.26069923670246E-19));
#7944=DIRECTION('center_axis',(-0.377681861983727,-0.843372107574981,-0.382204002193907));
#7945=DIRECTION('ref_axis',(0.592794689304909,-0.537329962094554,0.599892463836112));
#7946=DIRECTION('center_axis',(-0.0522650609395818,0.0520327192429072,0.997276771780618));
#7947=DIRECTION('ref_axis',(0.998629534754574,0.,0.0523359562429431));
#7948=DIRECTION('center_axis',(2.96465769266612E-15,-1.,0.));
#7949=DIRECTION('ref_axis',(0.,0.,1.));
#7950=DIRECTION('center_axis',(0.995216631131787,0.0976926666577189,1.18580395612125E-14));
#7951=DIRECTION('ref_axis',(0.0975341006448478,-0.993601284365854,0.0569524970297685));
#7952=DIRECTION('center_axis',(-6.60704473394009E-21,-1.,1.26069923670246E-19));
#7953=DIRECTION('ref_axis',(0.688354575693758,0.,0.725374371012284));
#7954=DIRECTION('',(6.60704473394009E-21,1.,-1.26069923670246E-19));
#7955=DIRECTION('',(-6.60704473394009E-21,-1.,1.26069923670246E-19));
#7956=DIRECTION('center_axis',(0.998629534754574,0.,-0.0523359562429438));
#7957=DIRECTION('ref_axis',(-0.0523359562429438,0.,-0.998629534754574));
#7958=DIRECTION('center_axis',(-1.01338750660366E-31,1.26069923670246E-19,
1.));
#7959=DIRECTION('ref_axis',(1.,0.,1.01338750660366E-31));
#7960=DIRECTION('center_axis',(-0.998629534754574,0.,-0.0523359562429438));
#7961=DIRECTION('ref_axis',(-0.0523359562429438,0.,0.998629534754574));
#10631=CARTESIAN_POINT('',(0.,0.,0.));
#10632=CARTESIAN_POINT('Origin',(9.,-1.,0.8));
#10633=CARTESIAN_POINT('',(8.85,-1.,0.9));
#10634=CARTESIAN_POINT('Origin',(9.,-1.,0.9));
#10635=CARTESIAN_POINT('',(8.85,-1.,0.7));
#10636=CARTESIAN_POINT('',(8.85,-1.,0.8));
#10637=CARTESIAN_POINT('Origin',(9.,-1.,0.7));
#10638=CARTESIAN_POINT('Origin',(3.,-1.,0.8));
#10639=CARTESIAN_POINT('',(2.85,-1.,0.9));
#10640=CARTESIAN_POINT('Origin',(3.,-1.,0.9));
#10641=CARTESIAN_POINT('',(2.85,-1.,0.7));
#10642=CARTESIAN_POINT('',(2.85,-1.,0.8));
#10643=CARTESIAN_POINT('Origin',(3.,-1.,0.7));
#10644=CARTESIAN_POINT('Origin',(3.,1.,0.8));
#10645=CARTESIAN_POINT('',(2.85,1.,0.9));
#10646=CARTESIAN_POINT('Origin',(3.,1.,0.9));
#10647=CARTESIAN_POINT('',(2.85,1.,0.7));
#10648=CARTESIAN_POINT('',(2.85,1.,0.8));
#10649=CARTESIAN_POINT('Origin',(3.,1.,0.7));
#10650=CARTESIAN_POINT('Origin',(9.,1.,0.8));
#10651=CARTESIAN_POINT('',(8.85,1.,0.9));
#10652=CARTESIAN_POINT('Origin',(9.,1.,0.9));
#10653=CARTESIAN_POINT('',(8.85,1.,0.7));
#10654=CARTESIAN_POINT('',(8.85,1.,0.8));
#10655=CARTESIAN_POINT('Origin',(9.,1.,0.7));
#10656=CARTESIAN_POINT('Origin',(10.1732050807569,0.3,0.9));
#10657=CARTESIAN_POINT('',(10.1732050807569,0.3,0.9));
#10658=CARTESIAN_POINT('',(10.3464101615138,0.,0.9));
#10659=CARTESIAN_POINT('',(9.72652155859676,1.07367855528516,0.9));
#10660=CARTESIAN_POINT('',(10.1732050807569,0.3,0.6));
#10661=CARTESIAN_POINT('',(10.1732050807569,0.3,0.9));
#10662=CARTESIAN_POINT('',(10.3464101615138,0.,0.6));
#10663=CARTESIAN_POINT('',(10.3464101615138,0.,0.6));
#10664=CARTESIAN_POINT('',(10.3464101615138,0.,0.9));
#10665=CARTESIAN_POINT('Origin',(9.82679491924311,0.3,0.9));
#10666=CARTESIAN_POINT('',(9.82679491924311,0.3,0.9));
#10667=CARTESIAN_POINT('',(7.95345829022414,0.3,0.9));
#10668=CARTESIAN_POINT('',(9.82679491924311,0.3,0.6));
#10669=CARTESIAN_POINT('',(9.82679491924311,0.3,0.9));
#10670=CARTESIAN_POINT('',(10.1732050807569,0.3,0.6));
#10671=CARTESIAN_POINT('Origin',(9.65358983848622,5.55111512312578E-17,
0.9));
#10672=CARTESIAN_POINT('',(9.65358983848622,4.24230095489963E-17,0.9));
#10673=CARTESIAN_POINT('',(9.2069063163261,-0.773678555285165,0.9));
#10674=CARTESIAN_POINT('',(9.65358983848622,5.55111512312578E-17,0.6));
#10675=CARTESIAN_POINT('',(9.65358983848622,4.24230095489963E-17,0.9));
#10676=CARTESIAN_POINT('',(9.82679491924311,0.3,0.6));
#10677=CARTESIAN_POINT('Origin',(9.82679491924311,-0.3,0.9));
#10678=CARTESIAN_POINT('',(9.82679491924311,-0.3,0.9));
#10679=CARTESIAN_POINT('',(9.29350885670454,0.623678555285165,0.9));
#10680=CARTESIAN_POINT('',(9.82679491924311,-0.3,0.6));
#10681=CARTESIAN_POINT('',(9.82679491924311,-0.3,0.9));
#10682=CARTESIAN_POINT('',(9.65358983848622,4.24230095489963E-17,0.6));
#10683=CARTESIAN_POINT('Origin',(10.1732050807569,-0.3,0.9));
#10684=CARTESIAN_POINT('',(10.1732050807569,-0.3,0.9));
#10685=CARTESIAN_POINT('',(8.12666337098103,-0.3,0.9));
#10686=CARTESIAN_POINT('',(10.1732050807569,-0.3,0.6));
#10687=CARTESIAN_POINT('',(10.1732050807569,-0.3,0.9));
#10688=CARTESIAN_POINT('',(9.82679491924311,-0.3,0.6));
#10689=CARTESIAN_POINT('Origin',(10.3464101615138,0.,0.9));
#10690=CARTESIAN_POINT('',(9.8131240989752,-0.923678555285165,0.9));
#10691=CARTESIAN_POINT('',(10.1732050807569,-0.3,0.6));
#10692=CARTESIAN_POINT('Origin',(10.,5.55111512312578E-17,0.6));
#10693=CARTESIAN_POINT('',(9.83,-2.0818995585505E-17,0.6));
#10694=CARTESIAN_POINT('Origin',(10.,0.,0.6));
#10695=CARTESIAN_POINT('Origin',(2.17320508075689,0.3,0.9));
#10696=CARTESIAN_POINT('',(2.17320508075689,0.3,0.9));
#10697=CARTESIAN_POINT('',(2.34641016151378,0.,0.9));
#10698=CARTESIAN_POINT('',(2.72652155859676,-0.65837225228371,0.9));
#10699=CARTESIAN_POINT('',(2.17320508075689,0.3,0.6));
#10700=CARTESIAN_POINT('',(2.17320508075689,0.3,0.9));
#10701=CARTESIAN_POINT('',(2.34641016151378,0.,0.6));
#10702=CARTESIAN_POINT('',(2.34641016151378,0.,0.6));
#10703=CARTESIAN_POINT('',(2.34641016151378,0.,0.9));
#10704=CARTESIAN_POINT('Origin',(1.82679491924311,0.3,0.9));
#10705=CARTESIAN_POINT('',(1.82679491924311,0.3,0.9));
#10706=CARTESIAN_POINT('',(3.95345829022414,0.3,0.9));
#10707=CARTESIAN_POINT('',(1.82679491924311,0.3,0.6));
#10708=CARTESIAN_POINT('',(1.82679491924311,0.3,0.9));
#10709=CARTESIAN_POINT('',(2.17320508075689,0.3,0.6));
#10710=CARTESIAN_POINT('Origin',(1.65358983848622,5.55111512312578E-17,
0.9));
#10711=CARTESIAN_POINT('',(1.65358983848622,4.24230095489963E-17,0.9));
#10712=CARTESIAN_POINT('',(2.20690631632609,0.958372252283711,0.9));
#10713=CARTESIAN_POINT('',(1.65358983848622,5.55111512312578E-17,0.6));
#10714=CARTESIAN_POINT('',(1.65358983848622,4.24230095489963E-17,0.9));
#10715=CARTESIAN_POINT('',(1.82679491924311,0.3,0.6));
#10716=CARTESIAN_POINT('Origin',(1.82679491924311,-0.3,0.9));
#10717=CARTESIAN_POINT('',(1.82679491924311,-0.3,0.9));
#10718=CARTESIAN_POINT('',(2.29350885670453,-1.10837225228371,0.9));
#10719=CARTESIAN_POINT('',(1.82679491924311,-0.3,0.6));
#10720=CARTESIAN_POINT('',(1.82679491924311,-0.3,0.9));
#10721=CARTESIAN_POINT('',(1.65358983848622,4.24230095489963E-17,0.6));
#10722=CARTESIAN_POINT('Origin',(2.17320508075689,-0.3,0.9));
#10723=CARTESIAN_POINT('',(2.17320508075689,-0.3,0.9));
#10724=CARTESIAN_POINT('',(4.12666337098103,-0.3,0.9));
#10725=CARTESIAN_POINT('',(2.17320508075689,-0.3,0.6));
#10726=CARTESIAN_POINT('',(2.17320508075689,-0.3,0.9));
#10727=CARTESIAN_POINT('',(1.82679491924311,-0.3,0.6));
#10728=CARTESIAN_POINT('Origin',(2.34641016151378,0.,0.9));
#10729=CARTESIAN_POINT('',(2.8131240989752,0.80837225228371,0.9));
#10730=CARTESIAN_POINT('',(2.17320508075689,-0.3,0.6));
#10731=CARTESIAN_POINT('Origin',(2.,5.55111512312578E-17,0.6));
#10732=CARTESIAN_POINT('',(1.83,-2.0818995585505E-17,0.6));
#10733=CARTESIAN_POINT('Origin',(2.,0.,0.6));
#10734=CARTESIAN_POINT('Origin',(2.,0.,0.45));
#10735=CARTESIAN_POINT('',(1.83,-2.0818995585505E-17,0.32));
#10736=CARTESIAN_POINT('',(1.83,2.0818995585505E-17,0.45));
#10737=CARTESIAN_POINT('Origin',(2.,0.,0.32));
#10738=CARTESIAN_POINT('Origin',(10.,0.,0.45));
#10739=CARTESIAN_POINT('',(9.83,-2.0818995585505E-17,0.32));
#10740=CARTESIAN_POINT('',(9.83,2.0818995585505E-17,0.45));
#10741=CARTESIAN_POINT('Origin',(10.,0.,0.32));
#10742=CARTESIAN_POINT('Origin',(11.2,-0.62,0.32));
#10743=CARTESIAN_POINT('',(0.200274469199584,-0.62,0.));
#10744=CARTESIAN_POINT('',(0.217044958570157,-0.62,0.32));
#10745=CARTESIAN_POINT('',(0.223426876981161,-0.62,0.441774257530303));
#10746=CARTESIAN_POINT('',(0.,-0.62,0.));
#10747=CARTESIAN_POINT('',(8.63987299740311,-0.62,0.));
#10748=CARTESIAN_POINT('',(0.0167704893705732,-0.62,0.32));
#10749=CARTESIAN_POINT('',(0.0237009700302462,-0.62,0.452241448778892));
#10750=CARTESIAN_POINT('',(-0.1,-0.62,0.32));
#10751=CARTESIAN_POINT('Origin',(11.2,-0.62,0.32));
#10752=CARTESIAN_POINT('',(0.9,-0.62,0.32));
#10753=CARTESIAN_POINT('',(0.9,-0.62,0.));
#10754=CARTESIAN_POINT('',(0.9,-0.62,0.16));
#10755=CARTESIAN_POINT('',(1.1,-0.62,0.32));
#10756=CARTESIAN_POINT('',(-0.1,-0.62,0.32));
#10757=CARTESIAN_POINT('',(1.1,-0.62,0.));
#10758=CARTESIAN_POINT('',(1.1,-0.62,0.16));
#10759=CARTESIAN_POINT('',(8.63987299740311,-0.62,0.));
#10760=CARTESIAN_POINT('Origin',(11.2,-0.62,0.32));
#10761=CARTESIAN_POINT('',(3.9,-0.62,0.32));
#10762=CARTESIAN_POINT('',(3.9,-0.62,0.));
#10763=CARTESIAN_POINT('',(3.9,-0.62,0.16));
#10764=CARTESIAN_POINT('',(4.1,-0.62,0.32));
#10765=CARTESIAN_POINT('',(-0.1,-0.62,0.32));
#10766=CARTESIAN_POINT('',(4.1,-0.62,0.));
#10767=CARTESIAN_POINT('',(4.1,-0.62,0.16));
#10768=CARTESIAN_POINT('',(8.63987299740311,-0.62,0.));
#10769=CARTESIAN_POINT('Origin',(11.2,-0.62,0.32));
#10770=CARTESIAN_POINT('',(7.9,-0.62,0.32));
#10771=CARTESIAN_POINT('',(7.9,-0.62,0.));
#10772=CARTESIAN_POINT('',(7.9,-0.62,0.16));
#10773=CARTESIAN_POINT('',(8.1,-0.62,0.32));
#10774=CARTESIAN_POINT('',(-0.1,-0.62,0.32));
#10775=CARTESIAN_POINT('',(8.1,-0.62,0.));
#10776=CARTESIAN_POINT('',(8.1,-0.62,0.16));
#10777=CARTESIAN_POINT('',(8.63987299740311,-0.62,0.));
#10778=CARTESIAN_POINT('Origin',(-0.0999999999999996,0.62,0.32));
#10779=CARTESIAN_POINT('',(0.217044958570158,0.62,0.32));
#10780=CARTESIAN_POINT('',(0.200274469199586,0.62,0.));
#10781=CARTESIAN_POINT('',(0.207951231396534,0.62,0.146481348799182));
#10782=CARTESIAN_POINT('',(0.0167704893705736,0.62,0.32));
#10783=CARTESIAN_POINT('',(11.2,0.62,0.32));
#10784=CARTESIAN_POINT('',(0.,0.62,0.));
#10785=CARTESIAN_POINT('',(0.00822532444561912,0.62,0.156948540047771));
#10786=CARTESIAN_POINT('',(2.98987299740311,0.62,0.));
#10787=CARTESIAN_POINT('Origin',(-0.0999999999999996,0.62,0.32));
#10788=CARTESIAN_POINT('',(0.9,0.62,0.));
#10789=CARTESIAN_POINT('',(0.9,0.62,0.32));
#10790=CARTESIAN_POINT('',(0.9,0.62,0.16));
#10791=CARTESIAN_POINT('',(1.1,0.62,0.));
#10792=CARTESIAN_POINT('',(2.98987299740311,0.62,0.));
#10793=CARTESIAN_POINT('',(1.1,0.62,0.32));
#10794=CARTESIAN_POINT('',(1.1,0.62,0.16));
#10795=CARTESIAN_POINT('',(11.2,0.62,0.32));
#10796=CARTESIAN_POINT('Origin',(-0.0999999999999996,0.62,0.32));
#10797=CARTESIAN_POINT('',(3.9,0.62,0.));
#10798=CARTESIAN_POINT('',(3.9,0.62,0.32));
#10799=CARTESIAN_POINT('',(3.9,0.62,0.16));
#10800=CARTESIAN_POINT('',(4.1,0.62,0.));
#10801=CARTESIAN_POINT('',(2.98987299740311,0.62,0.));
#10802=CARTESIAN_POINT('',(4.1,0.62,0.32));
#10803=CARTESIAN_POINT('',(4.1,0.62,0.16));
#10804=CARTESIAN_POINT('',(11.2,0.62,0.32));
#10805=CARTESIAN_POINT('Origin',(5.55,0.,0.32));
#10806=CARTESIAN_POINT('',(1.6,-4.89858719658941E-17,0.32));
#10807=CARTESIAN_POINT('Origin',(2.,0.,0.32));
#10808=CARTESIAN_POINT('Origin',(5.55,0.,0.32));
#10809=CARTESIAN_POINT('',(9.6,-4.89858719658942E-17,0.32));
#10810=CARTESIAN_POINT('Origin',(10.,0.,0.32));
#10811=CARTESIAN_POINT('Origin',(5.55,0.,0.32));
#10812=CARTESIAN_POINT('',(0.217044958570157,-0.7,0.32));
#10813=CARTESIAN_POINT('',(0.0167704893705731,-0.7,0.32));
#10814=CARTESIAN_POINT('Origin',(5.55,0.,0.32));
#10815=CARTESIAN_POINT('',(0.9,0.724814814814815,0.32));
#10816=CARTESIAN_POINT('',(1.1,-0.724814814814815,0.32));
#10817=CARTESIAN_POINT('Origin',(5.55,0.,0.32));
#10818=CARTESIAN_POINT('',(3.9,0.883148148148148,0.32));
#10819=CARTESIAN_POINT('',(4.1,-0.883148148148148,0.32));
#10820=CARTESIAN_POINT('Origin',(5.55,0.,0.32));
#10821=CARTESIAN_POINT('',(7.9,0.62,0.32));
#10822=CARTESIAN_POINT('',(7.9,0.886851851851852,0.32));
#10823=CARTESIAN_POINT('',(8.1,0.62,0.32));
#10824=CARTESIAN_POINT('',(11.2,0.62,0.32));
#10825=CARTESIAN_POINT('',(8.1,-0.886851851851852,0.32));
#10826=CARTESIAN_POINT('Origin',(-0.0999999999999996,0.62,0.32));
#10827=CARTESIAN_POINT('',(7.9,0.62,0.));
#10828=CARTESIAN_POINT('',(7.9,0.62,0.16));
#10829=CARTESIAN_POINT('',(8.1,0.62,0.));
#10830=CARTESIAN_POINT('',(2.98987299740311,0.62,0.));
#10831=CARTESIAN_POINT('',(8.1,0.62,0.16));
#10832=CARTESIAN_POINT('Origin',(11.2,1.53779953703704,0.));
#10833=CARTESIAN_POINT('',(11.2,1.47592264243751,0.));
#10834=CARTESIAN_POINT('',(11.2,-1.47592264243751,0.));
#10835=CARTESIAN_POINT('',(11.2,1.53779953703704,0.));
#10836=CARTESIAN_POINT('',(11.2,-1.44160695250311,0.605635447211793));
#10837=CARTESIAN_POINT('Ctrl Pts',(11.2,-1.44160695250311,0.605635447211793));
#10838=CARTESIAN_POINT('Ctrl Pts',(11.2,-1.44733381480461,0.504614841520655));
#10839=CARTESIAN_POINT('Ctrl Pts',(11.2,-1.45305922122436,0.403593539811385));
#10840=CARTESIAN_POINT('Ctrl Pts',(11.2,-1.46449774781658,0.201715464978033));
#10841=CARTESIAN_POINT('Ctrl Pts',(11.2,-1.47021094199039,0.100857470386242));
#10842=CARTESIAN_POINT('Ctrl Pts',(11.2,-1.47592264243751,0.));
#10843=CARTESIAN_POINT('',(11.2,-1.3413305091784,0.7));
#10844=CARTESIAN_POINT('Ctrl Pts',(11.2,-1.34133050917871,0.7));
#10845=CARTESIAN_POINT('Ctrl Pts',(11.2,-1.34927184579059,0.7));
#10846=CARTESIAN_POINT('Ctrl Pts',(11.1999981201149,-1.35715077597425,0.699006225306896));
#10847=CARTESIAN_POINT('Ctrl Pts',(11.1999964866412,-1.36482619101963,0.697118463987577));
#10848=CARTESIAN_POINT('Ctrl Pts',(11.1999955714568,-1.36912648693643,0.696060810134936));
#10849=CARTESIAN_POINT('Ctrl Pts',(11.1999947385598,-1.37336294684024,0.694721504600825));
#10850=CARTESIAN_POINT('Ctrl Pts',(11.1999942054834,-1.37750904339755,0.693111246644731));
#10851=CARTESIAN_POINT('Ctrl Pts',(11.1999932489192,-1.38494889279378,0.690221763364053));
#10852=CARTESIAN_POINT('Ctrl Pts',(11.1999934335488,-1.39201911070639,0.686493604183975));
#10853=CARTESIAN_POINT('Ctrl Pts',(11.1999946360439,-1.39857284316731,0.682006025455124));
#10854=CARTESIAN_POINT('Ctrl Pts',(11.1999952980149,-1.40218065925828,0.679535622697003));
#10855=CARTESIAN_POINT('Ctrl Pts',(11.1999962427007,-1.40563167682227,0.676834205328214));
#10856=CARTESIAN_POINT('Ctrl Pts',(11.1999970766466,-1.40889738828709,0.673909521834337));
#10857=CARTESIAN_POINT('Ctrl Pts',(11.1999978839828,-1.41205889660265,0.671078159882768));
#10858=CARTESIAN_POINT('Ctrl Pts',(11.1999985961359,-1.41502771690814,0.668054510912379));
#10859=CARTESIAN_POINT('Ctrl Pts',(11.1999985943254,-1.41778154893794,0.664849526385156));
#10860=CARTESIAN_POINT('Ctrl Pts',(11.1999985909468,-1.42292039881534,0.658868793295219));
#10861=CARTESIAN_POINT('Ctrl Pts',(11.1999963776609,-1.42731355725865,0.652257958652517));
#10862=CARTESIAN_POINT('Ctrl Pts',(11.1999956369,-1.43089859237711,0.645180832176479));
#10863=CARTESIAN_POINT('Ctrl Pts',(11.1999955610412,-1.43126572346771,0.644456088045497));
#10864=CARTESIAN_POINT('Ctrl Pts',(11.1999954968237,-1.43162433912915,0.643726434786758));
#10865=CARTESIAN_POINT('Ctrl Pts',(11.1999954455063,-1.43197434355081,0.642992037678167));
#10866=CARTESIAN_POINT('Ctrl Pts',(11.1999949451572,-1.43538691836834,0.635831599341589));
#10867=CARTESIAN_POINT('Ctrl Pts',(11.1999960935741,-1.43794480573841,0.628305806294037));
#10868=CARTESIAN_POINT('Ctrl Pts',(11.1999977538348,-1.43959303921538,0.620581877990282));
#10869=CARTESIAN_POINT('Ctrl Pts',(11.1999988103007,-1.44064185190664,0.615666946856702));
#10870=CARTESIAN_POINT('Ctrl Pts',(11.1999999935832,-1.44132148083109,0.610671141596651));
#10871=CARTESIAN_POINT('Ctrl Pts',(11.1999999950647,-1.44160695392865,0.605635447210179));
#10872=CARTESIAN_POINT('',(11.2,1.34133050917871,0.7));
#10873=CARTESIAN_POINT('',(11.2,0.768899768518519,0.7));
#10874=CARTESIAN_POINT('',(11.2,1.44160695250311,0.605635447211793));
#10875=CARTESIAN_POINT('Ctrl Pts',(11.1999999950647,1.44160695392865,0.605635447210179));
#10876=CARTESIAN_POINT('Ctrl Pts',(11.1999999927383,1.44115867123275,0.613543073794128));
#10877=CARTESIAN_POINT('Ctrl Pts',(11.199997327584,1.43974095598264,0.62135504174347));
#10878=CARTESIAN_POINT('Ctrl Pts',(11.1999961426836,1.43743894790867,0.628911795513178));
#10879=CARTESIAN_POINT('Ctrl Pts',(11.1999954950047,1.43618064644969,0.633042395401645));
#10880=CARTESIAN_POINT('Ctrl Pts',(11.1999951984378,1.4346571631488,0.63709676955888));
#10881=CARTESIAN_POINT('Ctrl Pts',(11.1999953420225,1.43287614971348,0.641047046155727));
#10882=CARTESIAN_POINT('Ctrl Pts',(11.1999956050472,1.42961361303411,0.648283331988978));
#10883=CARTESIAN_POINT('Ctrl Pts',(11.1999975633633,1.42552584716917,0.655091209244077));
#10884=CARTESIAN_POINT('Ctrl Pts',(11.1999983488166,1.42067941835906,0.661308913390503));
#10885=CARTESIAN_POINT('Ctrl Pts',(11.1999985007599,1.41974189284539,0.662511707551344));
#10886=CARTESIAN_POINT('Ctrl Pts',(11.1999985958742,1.41877583892185,0.663692344451305));
#10887=CARTESIAN_POINT('Ctrl Pts',(11.1999985956185,1.41778154881703,0.664849526385225));
#10888=CARTESIAN_POINT('Ctrl Pts',(11.199998595152,1.41596832836708,0.666959801783445));
#10889=CARTESIAN_POINT('Ctrl Pts',(11.1999982799021,1.41406123008998,0.668992111776222));
#10890=CARTESIAN_POINT('Ctrl Pts',(11.1999978412043,1.41206657472189,0.670943322037058));
#10891=CARTESIAN_POINT('Ctrl Pts',(11.1999965906985,1.40638082038708,0.676505236328724));
#10892=CARTESIAN_POINT('Ctrl Pts',(11.1999945592311,1.40005057587654,0.681348449922958));
#10893=CARTESIAN_POINT('Ctrl Pts',(11.1999938793032,1.39324090595796,0.685420973467861));
#10894=CARTESIAN_POINT('Ctrl Pts',(11.1999934424014,1.38886521116801,0.68803785802621));
#10895=CARTESIAN_POINT('Ctrl Pts',(11.1999934711477,1.38429057260668,0.690335857752236));
#10896=CARTESIAN_POINT('Ctrl Pts',(11.1999939665515,1.37955471147715,0.692291686537622));
#10897=CARTESIAN_POINT('Ctrl Pts',(11.1999947349645,1.37220899016913,0.695325342464331));
#10898=CARTESIAN_POINT('Ctrl Pts',(11.1999966395725,1.36455954597093,0.697503651902993));
#10899=CARTESIAN_POINT('Ctrl Pts',(11.1999981885915,1.35675452105021,0.698758058199902));
#10900=CARTESIAN_POINT('Ctrl Pts',(11.1999991983045,1.35166689148409,0.699575730741489));
#10901=CARTESIAN_POINT('Ctrl Pts',(11.2,1.34651254223162,0.7));
#10902=CARTESIAN_POINT('Ctrl Pts',(11.2,1.34133050917871,0.7));
#10903=CARTESIAN_POINT('Ctrl Pts',(11.2,1.47592264243751,0.));
#10904=CARTESIAN_POINT('Ctrl Pts',(11.2,1.47021025951677,0.100869521536925));
#10905=CARTESIAN_POINT('Ctrl Pts',(11.2,1.4644963825062,0.20173956751342));
#10906=CARTESIAN_POINT('Ctrl Pts',(11.2,1.45305785520703,0.403617642353031));
#10907=CARTESIAN_POINT('Ctrl Pts',(11.2,1.44733313162379,0.50462689268162));
#10908=CARTESIAN_POINT('Ctrl Pts',(11.2,1.44160695250311,0.605635447211793));
#10909=CARTESIAN_POINT('Origin',(8.1,-1.7737037037037,0.));
#10910=CARTESIAN_POINT('',(8.1,1.69866351109718,0.));
#10911=CARTESIAN_POINT('',(8.1,-1.7737037037037,0.));
#10912=CARTESIAN_POINT('',(8.1,1.66641703131627,0.605314487869832));
#10913=CARTESIAN_POINT('Ctrl Pts',(8.1,1.66641703131627,0.605314487869832));
#10914=CARTESIAN_POINT('Ctrl Pts',(8.1,1.67178339996556,0.504592280948055));
#10915=CARTESIAN_POINT('Ctrl Pts',(8.1,1.67714947719849,0.403869246528492));
#10916=CARTESIAN_POINT('Ctrl Pts',(8.1,1.68789827452893,0.202098297941347));
#10917=CARTESIAN_POINT('Ctrl Pts',(8.1,1.69328107955938,0.101048748975501));
#10918=CARTESIAN_POINT('Ctrl Pts',(8.1,1.69866351109718,0.));
#10919=CARTESIAN_POINT('',(8.1,1.56644778183753,0.7));
#10920=CARTESIAN_POINT('Ctrl Pts',(8.0999999986552,1.56644778212326,0.7));
#10921=CARTESIAN_POINT('Ctrl Pts',(8.10000000155239,1.57436337254628,0.699999999341293));
#10922=CARTESIAN_POINT('Ctrl Pts',(8.09999905041684,1.58221543358893,0.699005989267703));
#10923=CARTESIAN_POINT('Ctrl Pts',(8.09999821745812,1.58986365929578,0.697118696434997));
#10924=CARTESIAN_POINT('Ctrl Pts',(8.099997748439,1.59417019217574,0.69605600700222));
#10925=CARTESIAN_POINT('Ctrl Pts',(8.09999731997616,1.59841215407948,0.694709061504878));
#10926=CARTESIAN_POINT('Ctrl Pts',(8.09999704681388,1.60256279759721,0.693088866918468));
#10927=CARTESIAN_POINT('Ctrl Pts',(8.09999655811104,1.60998853482381,0.690190246691698));
#10928=CARTESIAN_POINT('Ctrl Pts',(8.09999665589197,1.61704187682962,0.686451534538094));
#10929=CARTESIAN_POINT('Ctrl Pts',(8.09999726576867,1.62357667434142,0.681954089017224));
#10930=CARTESIAN_POINT('Ctrl Pts',(8.09999760196939,1.62717904774802,0.679474826559159));
#10931=CARTESIAN_POINT('Ctrl Pts',(8.09999808150314,1.6306235748906,0.676764109620253));
#10932=CARTESIAN_POINT('Ctrl Pts',(8.09999850764167,1.63388182210815,0.673830012183301));
#10933=CARTESIAN_POINT('Ctrl Pts',(8.09999892160867,1.637047006066,0.670979719520364));
#10934=CARTESIAN_POINT('Ctrl Pts',(8.09999928906958,1.640017230617,0.667935813742119));
#10935=CARTESIAN_POINT('Ctrl Pts',(8.09999928944056,1.64277007752663,0.664709670235875));
#10936=CARTESIAN_POINT('Ctrl Pts',(8.09999929012967,1.64788359851353,0.658716982277737));
#10937=CARTESIAN_POINT('Ctrl Pts',(8.09999816327153,1.65225000627493,0.652096887528603));
#10938=CARTESIAN_POINT('Ctrl Pts',(8.09999778355904,1.65580927004486,0.645014643130784));
#10939=CARTESIAN_POINT('Ctrl Pts',(8.09999774450894,1.65617530914943,0.644286296325024));
#10940=CARTESIAN_POINT('Ctrl Pts',(8.09999771143612,1.65653277094855,0.643553041785202));
#10941=CARTESIAN_POINT('Ctrl Pts',(8.0999976850083,1.65688156115921,0.642815048027137));
#10942=CARTESIAN_POINT('Ctrl Pts',(8.09999742811004,1.66027206465027,0.635641192980042));
#10943=CARTESIAN_POINT('Ctrl Pts',(8.09999800724182,1.66280786743682,0.628104262855387));
#10944=CARTESIAN_POINT('Ctrl Pts',(8.09999885110511,1.66443535430957,0.620372450280339));
#10945=CARTESIAN_POINT('Ctrl Pts',(8.09999939164969,1.6654778563549,0.615419764910946));
#10946=CARTESIAN_POINT('Ctrl Pts',(8.1,1.66614680274328,0.610386449940169));
#10947=CARTESIAN_POINT('Ctrl Pts',(8.1,1.66641703131627,0.605314487869832));
#10948=CARTESIAN_POINT('',(8.1,-1.56644778183827,0.7));
#10949=CARTESIAN_POINT('',(8.1,-0.886851851851852,0.7));
#10950=CARTESIAN_POINT('',(8.1,-1.66641703131627,0.605314487869832));
#10951=CARTESIAN_POINT('Ctrl Pts',(8.1,-1.66641703131627,0.605314487869832));
#10952=CARTESIAN_POINT('Ctrl Pts',(8.1,-1.66599546653325,0.613226902778437));
#10953=CARTESIAN_POINT('Ctrl Pts',(8.09999864563672,-1.66460605882141,0.621047760783158));
#10954=CARTESIAN_POINT('Ctrl Pts',(8.09999804140045,-1.66233302739118,0.628616817026045));
#10955=CARTESIAN_POINT('Ctrl Pts',(8.09999770486592,-1.66106704316887,0.632832467392296));
#10956=CARTESIAN_POINT('Ctrl Pts',(8.0999975536836,-1.65952595995304,0.636970042829054));
#10957=CARTESIAN_POINT('Ctrl Pts',(8.09999763427866,-1.65771765414013,0.640999885518982));
#10958=CARTESIAN_POINT('Ctrl Pts',(8.09999777898787,-1.65447082344915,0.64823550729937));
#10959=CARTESIAN_POINT('Ctrl Pts',(8.09999878245444,-1.65040085231772,0.655045563401426));
#10960=CARTESIAN_POINT('Ctrl Pts',(8.09999917121848,-1.64557198994432,0.661267087195486));
#10961=CARTESIAN_POINT('Ctrl Pts',(8.09999924425118,-1.6446648462537,0.662435854416292));
#10962=CARTESIAN_POINT('Ctrl Pts',(8.09999928944999,-1.64373079085321,0.663583781603691));
#10963=CARTESIAN_POINT('Ctrl Pts',(8.09999928890117,-1.64277007755202,0.664709670235858));
#10964=CARTESIAN_POINT('Ctrl Pts',(8.09999928782175,-1.64088054556816,0.666924069243459));
#10965=CARTESIAN_POINT('Ctrl Pts',(8.09999911129818,-1.63888792496677,0.66905326411728));
#10966=CARTESIAN_POINT('Ctrl Pts',(8.09999887085824,-1.63679941630975,0.671093569621172));
#10967=CARTESIAN_POINT('Ctrl Pts',(8.09999821641022,-1.6311147520694,0.676647030794692));
#10968=CARTESIAN_POINT('Ctrl Pts',(8.0999972000003,-1.62478663867955,0.681482189379454));
#10969=CARTESIAN_POINT('Ctrl Pts',(8.09999686812141,-1.6179789612855,0.685544965666037));
#10970=CARTESIAN_POINT('Ctrl Pts',(8.09999665686968,-1.61364565292072,0.68813105508359));
#10971=CARTESIAN_POINT('Ctrl Pts',(8.09999667786582,-1.6091170759025,0.690403516124292));
#10972=CARTESIAN_POINT('Ctrl Pts',(8.0999969341683,-1.60442977212996,0.692339085768374));
#10973=CARTESIAN_POINT('Ctrl Pts',(8.09999733452329,-1.59710801128849,0.695362524980696));
#10974=CARTESIAN_POINT('Ctrl Pts',(8.09999831212369,-1.58948382509795,0.697531565976904));
#10975=CARTESIAN_POINT('Ctrl Pts',(8.09999909563861,-1.58170429192971,0.698776637084609));
#10976=CARTESIAN_POINT('Ctrl Pts',(8.09999960249138,-1.57667174192468,0.69958206878261));
#10977=CARTESIAN_POINT('Ctrl Pts',(8.1000000005313,-1.5715735875011,0.699999999573449));
#10978=CARTESIAN_POINT('Ctrl Pts',(8.0999999986552,-1.56644778212326,0.7));
#10979=CARTESIAN_POINT('',(8.1,-1.69866351109718,0.));
#10980=CARTESIAN_POINT('Ctrl Pts',(8.1,-1.69866351109718,0.));
#10981=CARTESIAN_POINT('Ctrl Pts',(8.1,-1.69328105674055,0.101049177371948));
#10982=CARTESIAN_POINT('Ctrl Pts',(8.1,-1.68789822886868,0.202099155105557));
#10983=CARTESIAN_POINT('Ctrl Pts',(8.1,-1.67714943151225,0.403870104074094));
#10984=CARTESIAN_POINT('Ctrl Pts',(8.1,-1.67178337712185,0.50459270970527));
#10985=CARTESIAN_POINT('Ctrl Pts',(8.1,-1.66641703131627,0.605314487869832));
#10986=CARTESIAN_POINT('',(8.1,-1.7737037037037,0.));
#10987=CARTESIAN_POINT('Origin',(4.1,-1.7662962962963,0.));
#10988=CARTESIAN_POINT('',(4.1,1.70113889814581,0.));
#10989=CARTESIAN_POINT('',(4.1,-1.7662962962963,0.));
#10990=CARTESIAN_POINT('',(4.1,1.66887738702937,0.605315322680072));
#10991=CARTESIAN_POINT('Ctrl Pts',(4.1,1.66887738702937,0.605315322680072));
#10992=CARTESIAN_POINT('Ctrl Pts',(4.1,1.67424235111642,0.50466767694528));
#10993=CARTESIAN_POINT('Ctrl Pts',(4.1,1.67960699363804,0.404019058341251));
#10994=CARTESIAN_POINT('Ctrl Pts',(4.1,1.69036079691899,0.202247931921761));
#10995=CARTESIAN_POINT('Ctrl Pts',(4.1,1.6957500571643,0.101123491803998));
#10996=CARTESIAN_POINT('Ctrl Pts',(4.1,1.70113889814581,0.));
#10997=CARTESIAN_POINT('',(4.1,1.56887583540973,0.7));
#10998=CARTESIAN_POINT('Ctrl Pts',(4.1,1.56887583540973,0.7));
#10999=CARTESIAN_POINT('Ctrl Pts',(4.1,1.57679416129392,0.7));
#11000=CARTESIAN_POINT('Ctrl Pts',(4.10000107724674,1.58464912207822,0.699006028000541));
#11001=CARTESIAN_POINT('Ctrl Pts',(4.10000201939527,1.59230028572239,0.697118705459362));
#11002=CARTESIAN_POINT('Ctrl Pts',(4.10000255022779,1.59661116283941,0.696055335763773));
#11003=CARTESIAN_POINT('Ctrl Pts',(4.10000303435977,1.60085740028891,0.694707333985525));
#11004=CARTESIAN_POINT('Ctrl Pts',(4.10000334030352,1.60501217339351,0.693085708041268));
#11005=CARTESIAN_POINT('Ctrl Pts',(4.10000388718746,1.61243895913315,0.690187001388783));
#11006=CARTESIAN_POINT('Ctrl Pts',(4.10000376557609,1.61949349263125,0.686448444730844));
#11007=CARTESIAN_POINT('Ctrl Pts',(4.10000306534783,1.6260295229635,0.681951159450519));
#11008=CARTESIAN_POINT('Ctrl Pts',(4.10000267892397,1.62963645835533,0.679469313954069));
#11009=CARTESIAN_POINT('Ctrl Pts',(4.10000213012555,1.63308521926452,0.676755517937216));
#11010=CARTESIAN_POINT('Ctrl Pts',(4.1000016436875,1.63634725251217,0.673817835781739));
#11011=CARTESIAN_POINT('Ctrl Pts',(4.10000117237165,1.63950787692018,0.67097147916344));
#11012=CARTESIAN_POINT('Ctrl Pts',(4.10000075597222,1.64247408874941,0.667932078875657));
#11013=CARTESIAN_POINT('Ctrl Pts',(4.10000075698646,1.64522354659423,0.664710927554201));
#11014=CARTESIAN_POINT('Ctrl Pts',(4.1000007588733,1.65033845220459,0.658718515269377));
#11015=CARTESIAN_POINT('Ctrl Pts',(4.10000204656096,1.65470614797426,0.652098486008568));
#11016=CARTESIAN_POINT('Ctrl Pts',(4.10000248678323,1.65826650381873,0.645016049251367));
#11017=CARTESIAN_POINT('Ctrl Pts',(4.10000253228732,1.65863452415637,0.644283964909082));
#11018=CARTESIAN_POINT('Ctrl Pts',(4.10000257095464,1.65899387729575,0.643546919913709));
#11019=CARTESIAN_POINT('Ctrl Pts',(4.10000260201855,1.65934446736461,0.642805085364403));
#11020=CARTESIAN_POINT('Ctrl Pts',(4.10000290242009,1.66273482600052,0.635631222228741));
#11021=CARTESIAN_POINT('Ctrl Pts',(4.10000225562543,1.66527033938482,0.628094305374488));
#11022=CARTESIAN_POINT('Ctrl Pts',(4.10000130084992,1.66689736875237,0.62036252267401));
#11023=CARTESIAN_POINT('Ctrl Pts',(4.10000068968835,1.66793884687677,0.615413329558163));
#11024=CARTESIAN_POINT('Ctrl Pts',(4.09999999901039,1.66860722297681,0.610383627857512));
#11025=CARTESIAN_POINT('Ctrl Pts',(4.09999999630223,1.66887738567036,0.60531532268817));
#11026=CARTESIAN_POINT('',(4.1,-1.56887583540947,0.7));
#11027=CARTESIAN_POINT('',(4.1,-0.883148148148148,0.7));
#11028=CARTESIAN_POINT('',(4.1,-1.66887738702937,0.605315322680072));
#11029=CARTESIAN_POINT('Ctrl Pts',(4.09999999630223,-1.66887738567036,0.60531532268817));
#11030=CARTESIAN_POINT('Ctrl Pts',(4.10000000053001,-1.66845562780346,0.613227583070809));
#11031=CARTESIAN_POINT('Ctrl Pts',(4.10000153668442,-1.66706589531621,0.621048261667561));
#11032=CARTESIAN_POINT('Ctrl Pts',(4.10000221487211,-1.66479240287642,0.628617079688242));
#11033=CARTESIAN_POINT('Ctrl Pts',(4.10000259231836,-1.6635270876889,0.632829515245766));
#11034=CARTESIAN_POINT('Ctrl Pts',(4.10000275805793,-1.66198703315979,0.636963972243471));
#11035=CARTESIAN_POINT('Ctrl Pts',(4.10000266178038,-1.66018010017296,0.640990858692597));
#11036=CARTESIAN_POINT('Ctrl Pts',(4.10000248876893,-1.65693302887506,0.648227201990446));
#11037=CARTESIAN_POINT('Ctrl Pts',(4.10000134097948,-1.65286254930452,0.655037795911226));
#11038=CARTESIAN_POINT('Ctrl Pts',(4.100000893742,-1.6480330317196,0.661259713776781));
#11039=CARTESIAN_POINT('Ctrl Pts',(4.10000080951506,-1.647123502594,0.662431469633614));
#11040=CARTESIAN_POINT('Ctrl Pts',(4.10000075717637,-1.6461869221106,0.663582276554164));
#11041=CARTESIAN_POINT('Ctrl Pts',(4.10000075728519,-1.64522354661022,0.66471092755419));
#11042=CARTESIAN_POINT('Ctrl Pts',(4.10000075749815,-1.64333815989002,0.666919768869269));
#11043=CARTESIAN_POINT('Ctrl Pts',(4.1000009568795,-1.64135017761634,0.669043797975229));
#11044=CARTESIAN_POINT('Ctrl Pts',(4.10000122972053,-1.63926675509047,0.671079366787198));
#11045=CARTESIAN_POINT('Ctrl Pts',(4.10000197419082,-1.6335819569127,0.676633591976433));
#11046=CARTESIAN_POINT('Ctrl Pts',(4.10000313643093,-1.62725355063421,0.681469444454218));
#11047=CARTESIAN_POINT('Ctrl Pts',(4.1000035230587,-1.62044557755217,0.685533082105531));
#11048=CARTESIAN_POINT('Ctrl Pts',(4.10000376939409,-1.61610795658125,0.688122181633714));
#11049=CARTESIAN_POINT('Ctrl Pts',(4.10000375220654,-1.61157469281532,0.690397125746379));
#11050=CARTESIAN_POINT('Ctrl Pts',(4.10000346632868,-1.60688245467732,0.692334655286926));
#11051=CARTESIAN_POINT('Ctrl Pts',(4.10000302008581,-1.59955807566073,0.695359054367588));
#11052=CARTESIAN_POINT('Ctrl Pts',(4.1000019139068,-1.59193114173487,0.69752894708864));
#11053=CARTESIAN_POINT('Ctrl Pts',(4.10000102635309,-1.58414888227482,0.698774888159427));
#11054=CARTESIAN_POINT('Ctrl Pts',(4.10000045177616,-1.57911086966871,0.699581474839467));
#11055=CARTESIAN_POINT('Ctrl Pts',(4.1,-1.57400716417114,0.7));
#11056=CARTESIAN_POINT('Ctrl Pts',(4.1,-1.56887583540973,0.7));
#11057=CARTESIAN_POINT('',(4.1,-1.70113889814582,0.));
#11058=CARTESIAN_POINT('Ctrl Pts',(4.1,-1.70113889814582,0.));
#11059=CARTESIAN_POINT('Ctrl Pts',(4.1,-1.69575004793467,0.101123665001254));
#11060=CARTESIAN_POINT('Ctrl Pts',(4.1,-1.69036077845691,0.202248278345555));
#11061=CARTESIAN_POINT('Ctrl Pts',(4.1,-1.67960697517202,0.404019404791024));
#11062=CARTESIAN_POINT('Ctrl Pts',(4.1,-1.67424234188296,0.504667850166609));
#11063=CARTESIAN_POINT('Ctrl Pts',(4.1,-1.66887738702937,0.605315322680072));
#11064=CARTESIAN_POINT('',(4.1,-1.7662962962963,0.));
#11065=CARTESIAN_POINT('Origin',(1.1,-1.44962962962963,0.));
#11066=CARTESIAN_POINT('',(1.1,1.39262953588351,0.));
#11067=CARTESIAN_POINT('',(1.1,-1.44962962962963,0.));
#11068=CARTESIAN_POINT('',(1.10000000000005,1.35674377243284,0.605845626926786));
#11069=CARTESIAN_POINT('Ctrl Pts',(1.10000000000005,1.35674377243284,0.605845626926786));
#11070=CARTESIAN_POINT('Ctrl Pts',(1.10000000000005,1.36273568520883,0.504787121979256));
#11071=CARTESIAN_POINT('Ctrl Pts',(1.1,1.36872466312622,0.403727404115485));
#11072=CARTESIAN_POINT('Ctrl Pts',(1.1,1.38068651056748,0.201779555185378));
#11073=CARTESIAN_POINT('Ctrl Pts',(1.1,1.38665951284069,0.10088935150083));
#11074=CARTESIAN_POINT('Ctrl Pts',(1.1,1.39262953588351,0.));
#11075=CARTESIAN_POINT('',(1.1,1.25565664448622,0.7));
#11076=CARTESIAN_POINT('Ctrl Pts',(1.1,1.25565664448621,0.7));
#11077=CARTESIAN_POINT('Ctrl Pts',(1.1,1.26365753466764,0.700000000000001));
#11078=CARTESIAN_POINT('Ctrl Pts',(1.10000312127109,1.27160078819195,0.699008097631352));
#11079=CARTESIAN_POINT('Ctrl Pts',(1.10000579554281,1.27934333527045,0.697120485426804));
#11080=CARTESIAN_POINT('Ctrl Pts',(1.10000709386889,1.28310224676699,0.696204072889075));
#11081=CARTESIAN_POINT('Ctrl Pts',(1.10000828779753,1.28681383019745,0.695075712339665));
#11082=CARTESIAN_POINT('Ctrl Pts',(1.10000913303706,1.29046059826345,0.693742188764313));
#11083=CARTESIAN_POINT('Ctrl Pts',(1.10001087659788,1.29798315455626,0.69099139518989));
#11084=CARTESIAN_POINT('Ctrl Pts',(1.10001086910546,1.30515375246939,0.687398976275641));
#11085=CARTESIAN_POINT('Ctrl Pts',(1.10000899624477,1.31182501206943,0.683041610144935));
#11086=CARTESIAN_POINT('Ctrl Pts',(1.10000779407289,1.31610723164143,0.680244657298552));
#11087=CARTESIAN_POINT('Ctrl Pts',(1.10000585478529,1.32018349952736,0.677131483611404));
#11088=CARTESIAN_POINT('Ctrl Pts',(1.10000422180804,1.32400796947387,0.673713330684339));
#11089=CARTESIAN_POINT('Ctrl Pts',(1.10000291018178,1.3270798280974,0.670967830603965));
#11090=CARTESIAN_POINT('Ctrl Pts',(1.10000180047651,1.32997084712789,0.668041731908725));
#11091=CARTESIAN_POINT('Ctrl Pts',(1.10000182449184,1.33266034096938,0.664944387470286));
#11092=CARTESIAN_POINT('Ctrl Pts',(1.10000187074845,1.33784065079383,0.65897850512594));
#11093=CARTESIAN_POINT('Ctrl Pts',(1.10000564109429,1.34227630326151,0.652378581761819));
#11094=CARTESIAN_POINT('Ctrl Pts',(1.10000696187003,1.34590032739451,0.645305437365917));
#11095=CARTESIAN_POINT('Ctrl Pts',(1.100007110355,1.34630774940504,0.644510256482779));
#11096=CARTESIAN_POINT('Ctrl Pts',(1.10000723579819,1.34670486410349,0.643709073603569));
#11097=CARTESIAN_POINT('Ctrl Pts',(1.10000733566964,1.34709153749004,0.642902104572485));
#11098=CARTESIAN_POINT('Ctrl Pts',(1.10000822022419,1.35051627708745,0.63575483535061));
#11099=CARTESIAN_POINT('Ctrl Pts',(1.10000635568239,1.35308446649167,0.628241602461225));
#11100=CARTESIAN_POINT('Ctrl Pts',(1.10000361780323,1.35473867947858,0.620527690691125));
#11101=CARTESIAN_POINT('Ctrl Pts',(1.1000019043033,1.35577396762308,0.615699943921843));
#11102=CARTESIAN_POINT('Ctrl Pts',(1.09999998677418,1.35645041192828,0.610792997969602));
#11103=CARTESIAN_POINT('Ctrl Pts',(1.09999997754868,1.35674374570294,0.605845627052288));
#11104=CARTESIAN_POINT('',(1.1,-1.25565664448622,0.7));
#11105=CARTESIAN_POINT('',(1.1,-0.724814814814815,0.7));
#11106=CARTESIAN_POINT('',(1.10000000000005,-1.35674377243284,0.605845626926786));
#11107=CARTESIAN_POINT('Ctrl Pts',(1.09999997754868,-1.35674374570294,0.605845627052288));
#11108=CARTESIAN_POINT('Ctrl Pts',(1.09999999227748,-1.35627542940044,0.613744255356351));
#11109=CARTESIAN_POINT('Ctrl Pts',(1.1000044245081,-1.35483313756702,0.621542702113576));
#11110=CARTESIAN_POINT('Ctrl Pts',(1.10000632213307,-1.3525036790266,0.629082464357584));
#11111=CARTESIAN_POINT('Ctrl Pts',(1.1000073336739,-1.3512619466217,0.633101581650771));
#11112=CARTESIAN_POINT('Ctrl Pts',(1.10000777634458,-1.34976719347553,0.637047225321331));
#11113=CARTESIAN_POINT('Ctrl Pts',(1.10000752568741,-1.34802684471036,0.640893844816285));
#11114=CARTESIAN_POINT('Ctrl Pts',(1.10000705344834,-1.3447480208661,0.648140890909733));
#11115=CARTESIAN_POINT('Ctrl Pts',(1.10000374385205,-1.34063788586045,0.654954534019122));
#11116=CARTESIAN_POINT('Ctrl Pts',(1.10000230512149,-1.33576793982513,0.661175616324976));
#11117=CARTESIAN_POINT('Ctrl Pts',(1.10000200863552,-1.33476436716076,0.662457623989879));
#11118=CARTESIAN_POINT('Ctrl Pts',(1.10000181701501,-1.33372836971272,0.663714393476354));
#11119=CARTESIAN_POINT('Ctrl Pts',(1.10000180919237,-1.33266033853372,0.664944387472089));
#11120=CARTESIAN_POINT('Ctrl Pts',(1.10000179685332,-1.33097567746633,0.666884520904953));
#11121=CARTESIAN_POINT('Ctrl Pts',(1.10000223926429,-1.32921133126375,0.668758058859172));
#11122=CARTESIAN_POINT('Ctrl Pts',(1.10000288715521,-1.32737234926393,0.670562692084704));
#11123=CARTESIAN_POINT('Ctrl Pts',(1.10000489069569,-1.32168547392559,0.676143347135183));
#11124=CARTESIAN_POINT('Ctrl Pts',(1.10000845923633,-1.31535192007569,0.681005160308095));
#11125=CARTESIAN_POINT('Ctrl Pts',(1.1000097672184,-1.30853956043085,0.685101187995272));
#11126=CARTESIAN_POINT('Ctrl Pts',(1.10001062829021,-1.30405484229164,0.687797688271992));
#11127=CARTESIAN_POINT('Ctrl Pts',(1.10001067755751,-1.29936155475819,0.690161668140197));
#11128=CARTESIAN_POINT('Ctrl Pts',(1.10000992106221,-1.29450057597768,0.692169783635984));
#11129=CARTESIAN_POINT('Ctrl Pts',(1.10000876843985,-1.28709422081189,0.695229417764685));
#11130=CARTESIAN_POINT('Ctrl Pts',(1.100005676647,-1.27938091857402,0.69743146309387));
#11131=CARTESIAN_POINT('Ctrl Pts',(1.10000309801581,-1.2715114871423,0.698709794160748));
#11132=CARTESIAN_POINT('Ctrl Pts',(1.10000138449209,-1.26628217885177,0.699559256705032));
#11133=CARTESIAN_POINT('Ctrl Pts',(1.1,-1.26098326598685,0.700000000000001));
#11134=CARTESIAN_POINT('Ctrl Pts',(1.1,-1.25565664448621,0.7));
#11135=CARTESIAN_POINT('',(1.1,-1.39262953588351,0.));
#11136=CARTESIAN_POINT('Ctrl Pts',(1.1,-1.39262953588351,0.));
#11137=CARTESIAN_POINT('Ctrl Pts',(1.1,-1.38665944902278,0.100890429980357));
#11138=CARTESIAN_POINT('Ctrl Pts',(1.1,-1.38068638286488,0.201781712214768));
#11139=CARTESIAN_POINT('Ctrl Pts',(1.1,-1.36872453529477,0.403729561179669));
#11140=CARTESIAN_POINT('Ctrl Pts',(1.10000000000005,-1.3627356212621,0.504788200493074));
#11141=CARTESIAN_POINT('Ctrl Pts',(1.10000000000005,-1.35674377243284,0.605845626926786));
#11142=CARTESIAN_POINT('',(1.1,-1.44962962962963,0.));
#11143=CARTESIAN_POINT('Origin',(0.199725906950915,-1.4,-0.0104671912485888));
#11144=CARTESIAN_POINT('',(0.200274469199584,1.15262458915154,1.38777878078145E-17));
#11145=CARTESIAN_POINT('',(0.200274469199585,-0.7,0.));
#11146=CARTESIAN_POINT('',(0.231993417893744,1.12115139781563,0.605233595624295));
#11147=CARTESIAN_POINT('Ctrl Pts',(0.200274469199584,1.15262458915154,-5.50774703622636E-17));
#11148=CARTESIAN_POINT('Ctrl Pts',(0.210847451072758,1.1421331482829,0.201744512318911));
#11149=CARTESIAN_POINT('Ctrl Pts',(0.221420433966108,1.13164208276446,0.403489044103923));
#11150=CARTESIAN_POINT('Ctrl Pts',(0.231993417893744,1.12115139781563,0.605233595624295));
#11151=CARTESIAN_POINT('',(0.231993417893744,-1.12115139781563,0.605233595624295));
#11152=CARTESIAN_POINT('',(0.231993417893744,-0.7,0.605233595624295));
#11153=CARTESIAN_POINT('',(0.200274469199584,-1.15262458915154,1.38777878078145E-17));
#11154=CARTESIAN_POINT('Ctrl Pts',(0.231993417893744,-1.12115139781563,
0.605233595624295));
#11155=CARTESIAN_POINT('Ctrl Pts',(0.221420433966108,-1.13164208276446,
0.403489044103923));
#11156=CARTESIAN_POINT('Ctrl Pts',(0.210847451072758,-1.1421331482829,0.201744512318911));
#11157=CARTESIAN_POINT('Ctrl Pts',(0.200274469199584,-1.15262458915154,
-6.67868538251071E-17));
#11158=CARTESIAN_POINT('',(0.200274469199585,-0.7,0.));
#11159=CARTESIAN_POINT('Origin',(6.07974599480623,0.,0.));
#11160=CARTESIAN_POINT('Ctrl Pts',(8.1,-1.69866351109718,4.37041895728907E-16));
#11161=CARTESIAN_POINT('Ctrl Pts',(8.9524267631348,-1.65897367198627,1.20944032620455E-7));
#11162=CARTESIAN_POINT('Ctrl Pts',(9.80407798130771,-1.59837060538327,2.76830114922109E-8));
#11163=CARTESIAN_POINT('Ctrl Pts',(10.6537697771985,-1.52488560579501,1.03413542584124E-8));
#11164=CARTESIAN_POINT('Ctrl Pts',(10.8359404901627,-1.50913069933138,6.62336842220622E-9));
#11165=CARTESIAN_POINT('Ctrl Pts',(11.0180211259896,-1.49278349820154,3.93228299510406E-9));
#11166=CARTESIAN_POINT('Ctrl Pts',(11.2000000002909,-1.47592264092474,-3.0227174540096E-11));
#11167=CARTESIAN_POINT('Ctrl Pts',(11.2000000002909,1.47592264092474,-3.02272213335841E-11));
#11168=CARTESIAN_POINT('Ctrl Pts',(10.4240589919717,1.54781576943643,1.68591524001238E-8));
#11169=CARTESIAN_POINT('Ctrl Pts',(9.64626799696257,1.61037563220813,6.17878738288937E-8));
#11170=CARTESIAN_POINT('Ctrl Pts',(8.86753211358286,1.65747704847969,5.27022751808308E-8));
#11171=CARTESIAN_POINT('Ctrl Pts',(8.61177933690776,1.67294611604661,4.97183789310355E-8));
#11172=CARTESIAN_POINT('Ctrl Pts',(8.35592462822135,1.68674740550612,3.63007687033005E-8));
#11173=CARTESIAN_POINT('Ctrl Pts',(8.1,1.69866351109718,3.71000138306103E-16));
#11174=CARTESIAN_POINT('',(7.9,1.70758761671949,0.));
#11175=CARTESIAN_POINT('',(7.9,1.7737037037037,0.));
#11176=CARTESIAN_POINT('Ctrl Pts',(7.90000000036908,1.70758761645525,-3.06814577203155E-11));
#11177=CARTESIAN_POINT('Ctrl Pts',(7.26247716501442,1.73478515342832,3.65175246633048E-8));
#11178=CARTESIAN_POINT('Ctrl Pts',(6.624575449312,1.74993328406844,-3.04558542439636E-7));
#11179=CARTESIAN_POINT('Ctrl Pts',(5.98677261990733,1.74972113442148,-3.1918790057331E-7));
#11180=CARTESIAN_POINT('Ctrl Pts',(5.35540610719671,1.74951112565922,-3.33669628155763E-7));
#11181=CARTESIAN_POINT('Ctrl Pts',(4.72663057529054,1.73425216511322,1.21151810208783E-7));
#11182=CARTESIAN_POINT('Ctrl Pts',(4.10000000045307,1.7011388979176,-4.27317258673188E-11));
#11183=CARTESIAN_POINT('',(3.9,1.68995649764597,0.));
#11184=CARTESIAN_POINT('',(3.9,1.7662962962963,0.));
#11185=CARTESIAN_POINT('Ctrl Pts',(3.9,1.68995649764597,-1.6113354923472E-17));
#11186=CARTESIAN_POINT('Ctrl Pts',(2.96252047830716,1.63464572816558,-1.61179993858831E-17));
#11187=CARTESIAN_POINT('Ctrl Pts',(2.02971500398675,1.53866944530133,-1.61823222708931E-17));
#11188=CARTESIAN_POINT('Ctrl Pts',(1.1,1.39262953588351,-1.60717230190728E-17));
#11189=CARTESIAN_POINT('',(0.9,1.3604297237941,0.));
#11190=CARTESIAN_POINT('',(0.9,1.44962962962963,0.));
#11191=CARTESIAN_POINT('',(0.28146619846596,1.25073018526678,0.));
#11192=CARTESIAN_POINT('Ctrl Pts',(0.899999999999963,1.36042972379409,2.53412200078296E-14));
#11193=CARTESIAN_POINT('Ctrl Pts',(0.693681964344164,1.32640030945436,-1.68820282978727E-7));
#11194=CARTESIAN_POINT('Ctrl Pts',(0.487510176034459,1.28986876146525,1.95094241611213E-11));
#11195=CARTESIAN_POINT('Ctrl Pts',(0.281466198465954,1.25073018526678,9.09211941846344E-16));
#11196=CARTESIAN_POINT('Ctrl Pts',(0.28146619846596,1.25073018526678,4.90059381963448E-17));
#11197=CARTESIAN_POINT('Ctrl Pts',(0.273672142824666,1.24924968434803,-1.60851827685828E-11));
#11198=CARTESIAN_POINT('Ctrl Pts',(0.266112037439191,1.2468180315926,-2.29735811958388E-6));
#11199=CARTESIAN_POINT('Ctrl Pts',(0.258922416881026,1.24354471831116,-3.39045428380668E-6));
#11200=CARTESIAN_POINT('Ctrl Pts',(0.254316658841251,1.24144779416325,-4.09070493067818E-6));
#11201=CARTESIAN_POINT('Ctrl Pts',(0.249862973385875,1.23900427835211,-4.3601744978078E-6));
#11202=CARTESIAN_POINT('Ctrl Pts',(0.245601965247185,1.23623285256398,-4.0505643599354E-6));
#11203=CARTESIAN_POINT('Ctrl Pts',(0.238945660500109,1.23190348870705,-3.5669089987193E-6));
#11204=CARTESIAN_POINT('Ctrl Pts',(0.232836306411817,1.22682685988243,-1.47564048465526E-6));
#11205=CARTESIAN_POINT('Ctrl Pts',(0.227416445112993,1.2210931256102,-3.43092614100725E-7));
#11206=CARTESIAN_POINT('Ctrl Pts',(0.225957664245637,1.21954986437275,-3.82620891408318E-8));
#11207=CARTESIAN_POINT('Ctrl Pts',(0.224549002474426,1.21795876469157,1.76022586487844E-7));
#11208=CARTESIAN_POINT('Ctrl Pts',(0.223193686986583,1.21632111005909,2.01577349231486E-7));
#11209=CARTESIAN_POINT('Ctrl Pts',(0.221344954485829,1.21408724984631,2.36435595047204E-7));
#11210=CARTESIAN_POINT('Ctrl Pts',(0.219595448227346,1.21176677459781,-7.7718209010198E-8));
#11211=CARTESIAN_POINT('Ctrl Pts',(0.217948412504407,1.20936721934621,-5.08402878561E-7));
#11212=CARTESIAN_POINT('Ctrl Pts',(0.213467776427723,1.20283941082417,-1.68004793834142E-6));
#11213=CARTESIAN_POINT('Ctrl Pts',(0.20978887558685,1.19579640990262,-3.43350901357988E-6));
#11214=CARTESIAN_POINT('Ctrl Pts',(0.206958221875648,1.18840352636746,-3.67425174897535E-6));
#11215=CARTESIAN_POINT('Ctrl Pts',(0.206193447398199,1.18640614723908,-3.7392946395744E-6));
#11216=CARTESIAN_POINT('Ctrl Pts',(0.205490847532167,1.18438308363371,-3.7149036306613E-6));
#11217=CARTESIAN_POINT('Ctrl Pts',(0.204851940804359,1.18233735619935,-3.6037364623937E-6));
#11218=CARTESIAN_POINT('Ctrl Pts',(0.202492508448082,1.17478264548698,-3.19320484275276E-6));
#11219=CARTESIAN_POINT('Ctrl Pts',(0.201019195184615,1.16698811697394,-1.36638523817118E-6));
#11220=CARTESIAN_POINT('Ctrl Pts',(0.200491965466086,1.15911075533121,-4.28455138775697E-7));
#11221=CARTESIAN_POINT('Ctrl Pts',(0.200347608840846,1.15695391685535,-1.71647870329038E-7));
#11222=CARTESIAN_POINT('Ctrl Pts',(0.200274469313241,1.15479080601565,-7.49035961899928E-12));
#11223=CARTESIAN_POINT('Ctrl Pts',(0.200274469199584,1.15262458915154,9.10729824887824E-18));
#11224=CARTESIAN_POINT('',(2.01407162049393E-18,1.15316892111334,2.77409355997279E-17));
#11225=CARTESIAN_POINT('',(0.,-1.4,0.));
#11226=CARTESIAN_POINT('',(0.243580684154574,1.44748675362873,2.77555756156289E-17));
#11227=CARTESIAN_POINT('Ctrl Pts',(0.243580684154575,1.44748675362873,-1.56125112837913E-16));
#11228=CARTESIAN_POINT('Ctrl Pts',(0.226022619058538,1.44415189332774,-6.74769223000006E-12));
#11229=CARTESIAN_POINT('Ctrl Pts',(0.208837776424359,1.43922483814223,-1.83343972289099E-6));
#11230=CARTESIAN_POINT('Ctrl Pts',(0.192216855517481,1.43283671850359,-2.37047811876899E-6));
#11231=CARTESIAN_POINT('Ctrl Pts',(0.175448307189507,1.42639185943196,-2.91228650265529E-6));
#11232=CARTESIAN_POINT('Ctrl Pts',(0.15925228528901,1.41845922211561,-2.09168970691363E-6));
#11233=CARTESIAN_POINT('Ctrl Pts',(0.143842215871583,1.4091253227419,-1.20497646612983E-7));
#11234=CARTESIAN_POINT('Ctrl Pts',(0.141154971457358,1.40749765525544,2.23243494969264E-7));
#11235=CARTESIAN_POINT('Ctrl Pts',(0.138491701959641,1.40582727297256,5.92673833856784E-7));
#11236=CARTESIAN_POINT('Ctrl Pts',(0.135853645420207,1.40411450883245,9.74556207071009E-7));
#11237=CARTESIAN_POINT('Ctrl Pts',(0.120686164410185,1.39426698768136,3.17018528370531E-6));
#11238=CARTESIAN_POINT('Ctrl Pts',(0.106484701177391,1.38310949089167,6.09567884445769E-6));
#11239=CARTESIAN_POINT('Ctrl Pts',(0.0934509959242968,1.37075049507673,
5.10227143121889E-6));
#11240=CARTESIAN_POINT('Ctrl Pts',(0.0918301157095608,1.36921352217444,
4.97873062758527E-6));
#11241=CARTESIAN_POINT('Ctrl Pts',(0.0902273306836925,1.36765791150105,
4.78983320752683E-6));
#11242=CARTESIAN_POINT('Ctrl Pts',(0.0886430622088043,1.36608382581751,
4.52250464763623E-6));
#11243=CARTESIAN_POINT('Ctrl Pts',(0.0755027622673366,1.35302798437193,
2.30521792157715E-6));
#11244=CARTESIAN_POINT('Ctrl Pts',(0.0636322991078783,1.33870385142449,
-4.95851449924696E-6));
#11245=CARTESIAN_POINT('Ctrl Pts',(0.0531272107863483,1.3233265665666,-1.07771754856876E-5));
#11246=CARTESIAN_POINT('Ctrl Pts',(0.0429100363670196,1.3083707283404,-1.64363639061758E-5));
#11247=CARTESIAN_POINT('Ctrl Pts',(0.0340657397255946,1.29253754778979,
-2.07072841115287E-5));
#11248=CARTESIAN_POINT('Ctrl Pts',(0.026663056477648,1.27603964904139,-2.15377272154938E-5));
#11249=CARTESIAN_POINT('Ctrl Pts',(0.0217318501145713,1.26504977678014,
-2.20909166714363E-5));
#11250=CARTESIAN_POINT('Ctrl Pts',(0.0174411483101006,1.25376411673155,
-2.12025196266096E-5));
#11251=CARTESIAN_POINT('Ctrl Pts',(0.01382286588119,1.24224013948332,-1.91534441809703E-5));
#11252=CARTESIAN_POINT('Ctrl Pts',(0.00842668188255806,1.22505366970124,
-1.60975223868617E-5));
#11253=CARTESIAN_POINT('Ctrl Pts',(0.00456091079961661,1.20745571355567,
-1.03588883906395E-5));
#11254=CARTESIAN_POINT('Ctrl Pts',(0.0023097402764219,1.18964331095195,
-5.71664032024866E-6));
#11255=CARTESIAN_POINT('Ctrl Pts',(0.00078319128522165,1.17756448131848,
-2.56866950429304E-6));
#11256=CARTESIAN_POINT('Ctrl Pts',(2.50028438421117E-9,1.16538650529032,
-1.91718613723104E-10));
#11257=CARTESIAN_POINT('Ctrl Pts',(-1.21430643318376E-17,1.15316892111333,
5.20417042793042E-18));
#11258=CARTESIAN_POINT('',(11.7295909468525,1.62672708026858,5.55111512312578E-17));
#11259=CARTESIAN_POINT('Ctrl Pts',(0.243580684154574,1.44748675362873,0.));
#11260=CARTESIAN_POINT('Ctrl Pts',(4.07225077172054,2.17467835246083,0.));
#11261=CARTESIAN_POINT('Ctrl Pts',(7.90092085928651,2.00057770191527,0.));
#11262=CARTESIAN_POINT('Ctrl Pts',(11.7295909468525,1.62672708026858,0.));
#11263=CARTESIAN_POINT('',(12.,1.32855945177638,-4.17473993839455E-17));
#11264=CARTESIAN_POINT('Ctrl Pts',(12.,1.32855945177638,2.42861286636753E-16));
#11265=CARTESIAN_POINT('Ctrl Pts',(11.9999999991614,1.34640852075174,-1.28298622986823E-11));
#11266=CARTESIAN_POINT('Ctrl Pts',(11.9983618543561,1.36418409382152,-2.22383001277967E-6));
#11267=CARTESIAN_POINT('Ctrl Pts',(11.9951861391139,1.38167870884165,-3.43465861540838E-6));
#11268=CARTESIAN_POINT('Ctrl Pts',(11.9919727904737,1.39938064150867,-4.65983598400874E-6));
#11269=CARTESIAN_POINT('Ctrl Pts',(11.9871848331028,1.41679645887758,-4.78742071954366E-6));
#11270=CARTESIAN_POINT('Ctrl Pts',(11.9808755917115,1.43370272794343,-3.5739118077222E-6));
#11271=CARTESIAN_POINT('Ctrl Pts',(11.9797611226834,1.43668906371449,-3.35955670324834E-6));
#11272=CARTESIAN_POINT('Ctrl Pts',(11.9785990681726,1.43965944485564,-3.11247275469786E-6));
#11273=CARTESIAN_POINT('Ctrl Pts',(11.9773895732386,1.44261255525912,-2.84353511336506E-6));
#11274=CARTESIAN_POINT('Ctrl Pts',(11.9705369081732,1.45934406518776,-1.31980853313606E-6));
#11275=CARTESIAN_POINT('Ctrl Pts',(11.9622259501015,1.47537448669426,1.24030492427686E-6));
#11276=CARTESIAN_POINT('Ctrl Pts',(11.9525330320198,1.49048867890869,8.79804099270529E-7));
#11277=CARTESIAN_POINT('Ctrl Pts',(11.9492586078121,1.49559449703792,7.58021100761347E-7));
#11278=CARTESIAN_POINT('Ctrl Pts',(11.9458260650319,1.50059560584699,2.73671093112169E-7));
#11279=CARTESIAN_POINT('Ctrl Pts',(11.9422371454499,1.50548309160802,-8.21070286398525E-7));
#11280=CARTESIAN_POINT('Ctrl Pts',(11.9335276940755,1.51734385321214,-3.47774636801117E-6));
#11281=CARTESIAN_POINT('Ctrl Pts',(11.923898315087,1.52853671512454,-9.61160164537397E-6));
#11282=CARTESIAN_POINT('Ctrl Pts',(11.9134480753511,1.53899918600446,-1.54908303532852E-5));
#11283=CARTESIAN_POINT('Ctrl Pts',(11.9006414429521,1.55182080751067,-2.26957483986032E-5));
#11284=CARTESIAN_POINT('Ctrl Pts',(11.8867118754531,1.56343792791748,-2.93307907620841E-5));
#11285=CARTESIAN_POINT('Ctrl Pts',(11.8718669715436,1.57375979462261,-3.2097080434168E-5));
#11286=CARTESIAN_POINT('Ctrl Pts',(11.8583226919989,1.58317731924447,-3.46210038525051E-5));
#11287=CARTESIAN_POINT('Ctrl Pts',(11.84401509256,1.59151672629289,-3.39892197405707E-5));
#11288=CARTESIAN_POINT('Ctrl Pts',(11.8290799708805,1.59867837245092,-3.04453078860132E-5));
#11289=CARTESIAN_POINT('Ctrl Pts',(11.8128282236205,1.60647136308226,-2.65889777530425E-5));
#11290=CARTESIAN_POINT('Ctrl Pts',(11.7959622791259,1.61280865470064,-1.93051308245346E-5));
#11291=CARTESIAN_POINT('Ctrl Pts',(11.7786680578171,1.61758555622507,-1.24065785496921E-5));
#11292=CARTESIAN_POINT('Ctrl Pts',(11.7626326571209,1.62201475420184,-6.0101616208217E-6));
#11293=CARTESIAN_POINT('Ctrl Pts',(11.7462278952123,1.62510256303752,-1.15598952599692E-10));
#11294=CARTESIAN_POINT('Ctrl Pts',(11.7295909468525,1.62672708026857,-1.01481323344643E-16));
#11295=CARTESIAN_POINT('',(12.,-1.32855945177638,-2.7831599589297E-17));
#11296=CARTESIAN_POINT('',(12.,1.6,0.));
#11297=CARTESIAN_POINT('',(11.7295909468525,-1.62672708026858,-2.77555756156289E-17));
#11298=CARTESIAN_POINT('Ctrl Pts',(11.7295909468525,-1.62672708026858,2.76688394418301E-16));
#11299=CARTESIAN_POINT('Ctrl Pts',(11.7473502233519,-1.62499297457843,3.63491969896433E-13));
#11300=CARTESIAN_POINT('Ctrl Pts',(11.7648769397846,-1.62163540491215,-2.46542030701863E-6));
#11301=CARTESIAN_POINT('Ctrl Pts',(11.7819744899096,-1.61677476461769,-3.87870576098494E-6));
#11302=CARTESIAN_POINT('Ctrl Pts',(11.799277951102,-1.61185558613358,-5.30901184740094E-6));
#11303=CARTESIAN_POINT('Ctrl Pts',(11.8161433440738,-1.60539638769883,-5.61072687595782E-6));
#11304=CARTESIAN_POINT('Ctrl Pts',(11.8323535184498,-1.59747214364331,-4.43708131311936E-6));
#11305=CARTESIAN_POINT('Ctrl Pts',(11.8351986841263,-1.59608130189932,-4.23108623901291E-6));
#11306=CARTESIAN_POINT('Ctrl Pts',(11.8380235988884,-1.59464521634493,-3.98890160078043E-6));
#11307=CARTESIAN_POINT('Ctrl Pts',(11.8408269920241,-1.59316415515964,-3.72087260345577E-6));
#11308=CARTESIAN_POINT('Ctrl Pts',(11.8568148563263,-1.58471760338924,-2.19229240409177E-6));
#11309=CARTESIAN_POINT('Ctrl Pts',(11.8719627312575,-1.57488689795395,5.08047814114288E-7));
#11310=CARTESIAN_POINT('Ctrl Pts',(11.8860639991294,-1.56376935451958,3.7910357452838E-7));
#11311=CARTESIAN_POINT('Ctrl Pts',(11.8908390360804,-1.5600046802233,3.35439876042474E-7));
#11312=CARTESIAN_POINT('Ctrl Pts',(11.8954938739134,-1.55609205312677,-6.31409548673105E-8));
#11313=CARTESIAN_POINT('Ctrl Pts',(11.9000197537765,-1.55203410647271,-1.07033715310124E-6));
#11314=CARTESIAN_POINT('Ctrl Pts',(11.9109521284419,-1.54223203603875,-3.50324446252274E-6));
#11315=CARTESIAN_POINT('Ctrl Pts',(11.9211333865357,-1.53158293117673,-9.37257606292525E-6));
#11316=CARTESIAN_POINT('Ctrl Pts',(11.9305114837192,-1.52019095639426,-1.50133174764804E-5));
#11317=CARTESIAN_POINT('Ctrl Pts',(11.9420285825687,-1.50620064502377,-2.19406264148308E-5));
#11318=CARTESIAN_POINT('Ctrl Pts',(11.9522379825693,-1.49120969914507,-2.8349487615449E-5));
#11319=CARTESIAN_POINT('Ctrl Pts',(11.9610699533786,-1.47543375940277,-3.10096306454085E-5));
#11320=CARTESIAN_POINT('Ctrl Pts',(11.9691383866925,-1.46102167397773,-3.34398002084833E-5));
#11321=CARTESIAN_POINT('Ctrl Pts',(11.976057247492,-1.44595309822982,-3.28127654573608E-5));
#11322=CARTESIAN_POINT('Ctrl Pts',(11.9817405815488,-1.43037347552767,-2.93737351251587E-5));
#11323=CARTESIAN_POINT('Ctrl Pts',(11.9879190063177,-1.41343666945002,-2.56351214921306E-5));
#11324=CARTESIAN_POINT('Ctrl Pts',(11.9925890154887,-1.39602986621001,-1.86015881889918E-5));
#11325=CARTESIAN_POINT('Ctrl Pts',(11.9956646601292,-1.37834843064327,-1.1951505214167E-5));
#11326=CARTESIAN_POINT('Ctrl Pts',(11.9985188379205,-1.36194017591583,-5.78027239782095E-6));
#11327=CARTESIAN_POINT('Ctrl Pts',(11.9999999979315,-1.34529424449622,-1.63143103698095E-10));
#11328=CARTESIAN_POINT('Ctrl Pts',(12.,-1.32855945177638,6.07153216591882E-17));
#11329=CARTESIAN_POINT('',(0.243580684154574,-1.44748675362873,-2.77555756156289E-17));
#11330=CARTESIAN_POINT('Ctrl Pts',(11.7295909468525,-1.62672708026858,0.));
#11331=CARTESIAN_POINT('Ctrl Pts',(7.90092085928651,-2.00057770191527,0.));
#11332=CARTESIAN_POINT('Ctrl Pts',(4.07225077172054,-2.17467835246083,0.));
#11333=CARTESIAN_POINT('Ctrl Pts',(0.243580684154574,-1.44748675362873,
0.));
#11334=CARTESIAN_POINT('',(-2.01407162049393E-18,-1.15316892111334,-2.77409355997279E-17));
#11335=CARTESIAN_POINT('Ctrl Pts',(-1.45716771982052E-16,-1.15316892111333,
-8.67361737988404E-17));
#11336=CARTESIAN_POINT('Ctrl Pts',(1.25998894435939E-9,-1.17105087373522,
-1.90287520688926E-11));
#11337=CARTESIAN_POINT('Ctrl Pts',(0.00163339464743996,-1.18886359576077,
-1.42965894531121E-6));
#11338=CARTESIAN_POINT('Ctrl Pts',(0.00480727841906161,-1.20639511031145,
-1.64093682142839E-6));
#11339=CARTESIAN_POINT('Ctrl Pts',(0.00800796397580062,-1.22407466931478,
-1.8539988284852E-6));
#11340=CARTESIAN_POINT('Ctrl Pts',(0.0127756311263789,-1.24146980201313,
-7.66483898132055E-7));
#11341=CARTESIAN_POINT('Ctrl Pts',(0.0190655400899108,-1.25835467436912,
1.24978183846727E-6));
#11342=CARTESIAN_POINT('Ctrl Pts',(0.0201762582672253,-1.26133632875492,
1.60582880463507E-6));
#11343=CARTESIAN_POINT('Ctrl Pts',(0.0213345630164365,-1.2643020159517,
1.98173645466097E-6));
#11344=CARTESIAN_POINT('Ctrl Pts',(0.022540357064946,-1.26725040777374,
2.36324320385681E-6));
#11345=CARTESIAN_POINT('Ctrl Pts',(0.0293845669280623,-1.28398578013164,
4.5287143794027E-6));
#11346=CARTESIAN_POINT('Ctrl Pts',(0.0376942987862453,-1.30001720705818,
7.20349268724091E-6));
#11347=CARTESIAN_POINT('Ctrl Pts',(0.0474014865253391,-1.31512615530125,
5.82569015349308E-6));
#11348=CARTESIAN_POINT('Ctrl Pts',(0.0485928463173857,-1.31698047129067,
5.65659292531477E-6));
#11349=CARTESIAN_POINT('Ctrl Pts',(0.049805315173965,-1.3188208685659,5.4220814195758E-6));
#11350=CARTESIAN_POINT('Ctrl Pts',(0.0510388164126442,-1.32064691964073,
5.10992468070797E-6));
#11351=CARTESIAN_POINT('Ctrl Pts',(0.0614399911345998,-1.33604461498541,
2.47774509321499E-6));
#11352=CARTESIAN_POINT('Ctrl Pts',(0.0733332132114129,-1.35042574344132,
-5.3152380038924E-6));
#11353=CARTESIAN_POINT('Ctrl Pts',(0.0865238753361435,-1.36365441213776,
-1.1550981620978E-5));
#11354=CARTESIAN_POINT('Ctrl Pts',(0.0993129767592984,-1.37648036310613,
-1.75968917362996E-5));
#11355=CARTESIAN_POINT('Ctrl Pts',(0.113220041589059,-1.38812080263946,
-2.21381304374214E-5));
#11356=CARTESIAN_POINT('Ctrl Pts',(0.128049501721596,-1.3984678073416,-2.30260298918279E-5));
#11357=CARTESIAN_POINT('Ctrl Pts',(0.137898881094142,-1.40534004502052,
-2.36157518704412E-5));
#11358=CARTESIAN_POINT('Ctrl Pts',(0.148156110210342,-1.41164106947418,
-2.26770903305374E-5));
#11359=CARTESIAN_POINT('Ctrl Pts',(0.158771208267938,-1.41732893485082,
-2.05010084084185E-5));
#11360=CARTESIAN_POINT('Ctrl Pts',(0.174640735071984,-1.42583226958806,
-1.72477751171679E-5));
#11361=CARTESIAN_POINT('Ctrl Pts',(0.191199787345415,-1.4329086754137,-1.11085100333009E-5));
#11362=CARTESIAN_POINT('Ctrl Pts',(0.208270835533445,-1.43843835369108,
-6.12965879291162E-6));
#11363=CARTESIAN_POINT('Ctrl Pts',(0.219822542278978,-1.44218019901621,
-2.76054936125183E-6));
#11364=CARTESIAN_POINT('Ctrl Pts',(0.231609382520684,-1.4452130041726,-1.10646384277296E-10));
#11365=CARTESIAN_POINT('Ctrl Pts',(0.243580684154575,-1.44748675362873,
-8.67361737988404E-18));
#11366=CARTESIAN_POINT('',(0.,-1.4,0.));
#11367=CARTESIAN_POINT('',(0.28146619846596,-1.25073018526678,-1.38777878078145E-17));
#11368=CARTESIAN_POINT('Ctrl Pts',(0.200274469199584,-1.15262458915154,
-4.38017677684144E-17));
#11369=CARTESIAN_POINT('Ctrl Pts',(0.200274469606231,-1.16056122076396,
-2.67994619525583E-11));
#11370=CARTESIAN_POINT('Ctrl Pts',(0.201251993787099,-1.16844573575355,
-2.06906772440415E-6));
#11371=CARTESIAN_POINT('Ctrl Pts',(0.203125250303271,-1.17612349127761,
-3.03593176598444E-6));
#11372=CARTESIAN_POINT('Ctrl Pts',(0.204328175564463,-1.18105381768481,
-3.65681052429326E-6));
#11373=CARTESIAN_POINT('Ctrl Pts',(0.205901645655995,-1.18589907428975,
-3.87486521964464E-6));
#11374=CARTESIAN_POINT('Ctrl Pts',(0.207834893326199,-1.19061551412018,
-3.56660141708203E-6));
#11375=CARTESIAN_POINT('Ctrl Pts',(0.210845733886816,-1.19796089907112,
-3.08651126907409E-6));
#11376=CARTESIAN_POINT('Ctrl Pts',(0.214691665920849,-1.20490884791767,
-1.13290501265697E-6));
#11377=CARTESIAN_POINT('Ctrl Pts',(0.219311372289421,-1.21130241743461,
-1.88024479619773E-7));
#11378=CARTESIAN_POINT('Ctrl Pts',(0.220549822002528,-1.21301640393121,
6.52788543367939E-8));
#11379=CARTESIAN_POINT('Ctrl Pts',(0.22184414018537,-1.21469042595737,2.26073670777299E-7));
#11380=CARTESIAN_POINT('Ctrl Pts',(0.223193686901845,-1.21632111014354,
1.99977909429435E-7));
#11381=CARTESIAN_POINT('Ctrl Pts',(0.225054776233359,-1.21856990146355,
1.63990609064731E-7));
#11382=CARTESIAN_POINT('Ctrl Pts',(0.227020882846909,-1.2207363067163,-2.2494482424301E-7));
#11383=CARTESIAN_POINT('Ctrl Pts',(0.229085096241527,-1.22281561536867,
-7.25033596408456E-7));
#11384=CARTESIAN_POINT('Ctrl Pts',(0.234663732853057,-1.22843504764494,
-2.07654770860772E-6));
#11385=CARTESIAN_POINT('Ctrl Pts',(0.240898147116973,-1.23336261820331,
-3.93931381885212E-6));
#11386=CARTESIAN_POINT('Ctrl Pts',(0.247634917667946,-1.2375211924479,-4.15647360184107E-6));
#11387=CARTESIAN_POINT('Ctrl Pts',(0.24944409362824,-1.23863798757926,-4.21479238469909E-6));
#11388=CARTESIAN_POINT('Ctrl Pts',(0.251289686356224,-1.23969909864123,
-4.17584617698396E-6));
#11389=CARTESIAN_POINT('Ctrl Pts',(0.253169062337335,-1.24070249413235,
-4.04352721072409E-6));
#11390=CARTESIAN_POINT('Ctrl Pts',(0.260147540238377,-1.24442829106235,
-3.55220190316667E-6));
#11391=CARTESIAN_POINT('Ctrl Pts',(0.267526846148503,-1.24732811138375,
-1.51439637010182E-6));
#11392=CARTESIAN_POINT('Ctrl Pts',(0.275164162321015,-1.24931347733136,
-4.73394739174148E-7));
#11393=CARTESIAN_POINT('Ctrl Pts',(0.277246452424842,-1.24985478107889,
-1.89568936341825E-7));
#11394=CARTESIAN_POINT('Ctrl Pts',(0.27934803608603,-1.25032783487679,-4.20368826828312E-12));
#11395=CARTESIAN_POINT('Ctrl Pts',(0.28146619846596,-1.25073018526678,1.2793585635329E-17));
#11396=CARTESIAN_POINT('',(0.9,-1.3604297237941,0.));
#11397=CARTESIAN_POINT('Ctrl Pts',(0.281466198465954,-1.25073018526678,
9.63150999927498E-16));
#11398=CARTESIAN_POINT('Ctrl Pts',(0.487510152792939,-1.28986875705046,
1.95065110193295E-11));
#11399=CARTESIAN_POINT('Ctrl Pts',(0.693681940810289,-1.32640030557063,
-1.68784634270162E-7));
#11400=CARTESIAN_POINT('Ctrl Pts',(0.899999999999961,-1.36042972379409,
2.52314774976951E-14));
#11401=CARTESIAN_POINT('',(0.9,1.44962962962963,0.));
#11402=CARTESIAN_POINT('',(3.9,-1.68995649764597,0.));
#11403=CARTESIAN_POINT('Ctrl Pts',(1.1,-1.39262953588351,-2.05019623674552E-17));
#11404=CARTESIAN_POINT('Ctrl Pts',(2.02971449277185,-1.53866936499954,-2.04062575199768E-17));
#11405=CARTESIAN_POINT('Ctrl Pts',(2.96251993741879,-1.63464569625347,-2.05230086706555E-17));
#11406=CARTESIAN_POINT('Ctrl Pts',(3.9,-1.68995649764597,-2.05203881127908E-17));
#11407=CARTESIAN_POINT('',(3.9,1.7662962962963,0.));
#11408=CARTESIAN_POINT('',(7.9,-1.70758761671949,0.));
#11409=CARTESIAN_POINT('Ctrl Pts',(4.10000000045307,-1.7011388979176,-4.27317380631109E-11));
#11410=CARTESIAN_POINT('Ctrl Pts',(4.72643887491804,-1.7342420350347,1.20853286712337E-7));
#11411=CARTESIAN_POINT('Ctrl Pts',(5.35502164560988,-1.74950180199062,-3.33551248611792E-7));
#11412=CARTESIAN_POINT('Ctrl Pts',(5.98619394951577,-1.74972093772735,-3.1920111515717E-7));
#11413=CARTESIAN_POINT('Ctrl Pts',(6.62418968669829,-1.74994244248134,-3.0469584628258E-7));
#11414=CARTESIAN_POINT('Ctrl Pts',(7.26228442347589,-1.73479337602516,3.6583895104054E-8));
#11415=CARTESIAN_POINT('Ctrl Pts',(7.90000000036908,-1.70758761645525,-3.06816097140251E-11));
#11416=CARTESIAN_POINT('',(7.9,1.7737037037037,0.));
#11417=CARTESIAN_POINT('',(11.4,-1.45718524058191,0.));
#11418=CARTESIAN_POINT('',(11.7095901160181,-1.42740242188993,1.38777878078145E-17));
#11419=CARTESIAN_POINT('Ctrl Pts',(11.4000000008084,-1.45718524050535,1.02728155843002E-16));
#11420=CARTESIAN_POINT('Ctrl Pts',(11.5032315878449,-1.44740895658952,-1.62414911853346E-10));
#11421=CARTESIAN_POINT('Ctrl Pts',(11.6064290066394,-1.43747657129068,3.17212713797596E-13));
#11422=CARTESIAN_POINT('Ctrl Pts',(11.7095901160181,-1.42740242188993,-1.31135713082882E-16));
#11423=CARTESIAN_POINT('',(11.7997255308004,-1.32801330383774,0.));
#11424=CARTESIAN_POINT('Ctrl Pts',(11.7095901160181,-1.42740242188993,-9.19403442267708E-17));
#11425=CARTESIAN_POINT('Ctrl Pts',(11.7174875668098,-1.42663119997609,-1.06723531187443E-12));
#11426=CARTESIAN_POINT('Ctrl Pts',(11.7252481284326,-1.42489860698852,-1.31351091787008E-6));
#11427=CARTESIAN_POINT('Ctrl Pts',(11.7327147629935,-1.4222933789697,-1.57347087725304E-6));
#11428=CARTESIAN_POINT('Ctrl Pts',(11.7375034508718,-1.42062252930751,-1.7401948673154E-6));
#11429=CARTESIAN_POINT('Ctrl Pts',(11.742171336984,-1.41859157258352,-1.52962160850981E-6));
#11430=CARTESIAN_POINT('Ctrl Pts',(11.7466731630754,-1.4162133745499,-1.06822103866601E-6));
#11431=CARTESIAN_POINT('Ctrl Pts',(11.7538080604269,-1.41244419322064,-3.36952074275293E-7));
#11432=CARTESIAN_POINT('Ctrl Pts',(11.7604421378066,-1.40785009750528,1.23525126371337E-6));
#11433=CARTESIAN_POINT('Ctrl Pts',(11.7664060685299,-1.40250292630552,-7.85770423176645E-8));
#11434=CARTESIAN_POINT('Ctrl Pts',(11.7700505374369,-1.39923534992309,-8.81437879006801E-7));
#11435=CARTESIAN_POINT('Ctrl Pts',(11.7734443324447,-1.39568546479044,-2.84121358692309E-6));
#11436=CARTESIAN_POINT('Ctrl Pts',(11.7765701913309,-1.39188797822873,-4.73246891796253E-6));
#11437=CARTESIAN_POINT('Ctrl Pts',(11.7816218974528,-1.38575085342217,-7.78893003218221E-6));
#11438=CARTESIAN_POINT('Ctrl Pts',(11.7859196635778,-1.3790373064984,-1.04294718165207E-5));
#11439=CARTESIAN_POINT('Ctrl Pts',(11.7894058487846,-1.37190723377291,-1.0649753115785E-5));
#11440=CARTESIAN_POINT('Ctrl Pts',(11.7909886780302,-1.36866997385604,-1.07497672177443E-5));
#11441=CARTESIAN_POINT('Ctrl Pts',(11.7924036476919,-1.36534638272796,-1.04045251440782E-5));
#11442=CARTESIAN_POINT('Ctrl Pts',(11.7936422141268,-1.36194984358789,-9.67400732978531E-6));
#11443=CARTESIAN_POINT('Ctrl Pts',(11.7963517531347,-1.35451943450186,-8.0758964348484E-6));
#11444=CARTESIAN_POINT('Ctrl Pts',(11.7981920551596,-1.34681816044402,-4.45435127417515E-6));
#11445=CARTESIAN_POINT('Ctrl Pts',(11.7990923524223,-1.33899256731255,-1.99131993767782E-6));
#11446=CARTESIAN_POINT('Ctrl Pts',(11.7995108157868,-1.33535518645399,-8.46488755312323E-7));
#11447=CARTESIAN_POINT('Ctrl Pts',(11.7997255306472,-1.33169069466208,-1.20180646731727E-11));
#11448=CARTESIAN_POINT('Ctrl Pts',(11.7997255308004,-1.32801330383774,1.56125112837913E-17));
#11449=CARTESIAN_POINT('',(11.7997255308004,1.32801330383774,-1.38777878078145E-17));
#11450=CARTESIAN_POINT('',(11.7997255308004,0.8,0.));
#11451=CARTESIAN_POINT('',(11.7095901160181,1.42740242188993,1.38777878078145E-17));
#11452=CARTESIAN_POINT('Ctrl Pts',(11.7997255308004,1.32801330383774,3.29597460435593E-17));
#11453=CARTESIAN_POINT('Ctrl Pts',(11.7997255306701,1.33594993357028,-3.19998942079111E-12));
#11454=CARTESIAN_POINT('Ctrl Pts',(11.7987557313351,1.34384388324515,-1.1738056914779E-6));
#11455=CARTESIAN_POINT('Ctrl Pts',(11.7968890528831,1.35153020534854,-1.35082478761126E-6));
#11456=CARTESIAN_POINT('Ctrl Pts',(11.7956902940742,1.35646627043222,-1.46450435604653E-6));
#11457=CARTESIAN_POINT('Ctrl Pts',(11.7941204989552,1.36131691981906,-1.21679535622301E-6));
#11458=CARTESIAN_POINT('Ctrl Pts',(11.7921880664813,1.36603565236267,-7.51718013047842E-7));
#11459=CARTESIAN_POINT('Ctrl Pts',(11.7891321441143,1.37349779167052,-1.62510435539431E-8));
#11460=CARTESIAN_POINT('Ctrl Pts',(11.7852081688769,1.38054242009704,1.47305143123643E-6));
#11461=CARTESIAN_POINT('Ctrl Pts',(11.7804707482717,1.38699431162271,4.31295153147674E-8));
#11462=CARTESIAN_POINT('Ctrl Pts',(11.7775673564694,1.39094843993989,-8.33217322910001E-7));
#11463=CARTESIAN_POINT('Ctrl Pts',(11.774357304366,1.39467961749964,-2.88177890715362E-6));
#11464=CARTESIAN_POINT('Ctrl Pts',(11.7708736118052,1.39816709864095,-4.85419454747415E-6));
#11465=CARTESIAN_POINT('Ctrl Pts',(11.7652557092992,1.40379111072049,-8.03496856102318E-6));
#11466=CARTESIAN_POINT('Ctrl Pts',(11.7589908599241,1.40872063947841,-1.07717451179728E-5));
#11467=CARTESIAN_POINT('Ctrl Pts',(11.7522324303862,1.41288246393566,-1.10093962897399E-5));
#11468=CARTESIAN_POINT('Ctrl Pts',(11.7491699691574,1.41476832010531,-1.11170836593312E-5));
#11469=CARTESIAN_POINT('Ctrl Pts',(11.7460056456443,1.41649603445901,-1.07652933077188E-5));
#11470=CARTESIAN_POINT('Ctrl Pts',(11.7427518690514,1.41805582819498,-1.00150721194158E-5));
#11471=CARTESIAN_POINT('Ctrl Pts',(11.7356218627913,1.421473806899,-8.37111113549047E-6));
#11472=CARTESIAN_POINT('Ctrl Pts',(11.7281378774234,1.42405291512428,-4.62166314666036E-6));
#11473=CARTESIAN_POINT('Ctrl Pts',(11.7204387731059,1.42570834923663,-2.06587013620581E-6));
#11474=CARTESIAN_POINT('Ctrl Pts',(11.7168648812537,1.42647679479109,-8.79481766934018E-7));
#11475=CARTESIAN_POINT('Ctrl Pts',(11.7132443218769,1.42704557200794,-8.45784208685192E-12));
#11476=CARTESIAN_POINT('Ctrl Pts',(11.7095901160181,1.42740242188993,2.53703308361608E-17));
#11477=CARTESIAN_POINT('',(11.4,1.45718524058191,0.));
#11478=CARTESIAN_POINT('Ctrl Pts',(11.7095901160181,1.42740242188993,-2.09644042577228E-16));
#11479=CARTESIAN_POINT('Ctrl Pts',(11.6064290073882,1.43747657121756,3.16925904777201E-13));
#11480=CARTESIAN_POINT('Ctrl Pts',(11.5032315885351,1.44740895652415,-1.62368751268212E-10));
#11481=CARTESIAN_POINT('Ctrl Pts',(11.4000000008083,1.45718524050537,-7.57963810214684E-17));
#11482=CARTESIAN_POINT('',(11.4,-1.53779953703704,0.));
#11483=CARTESIAN_POINT('Origin',(10.,0.,0.));
#11484=CARTESIAN_POINT('',(9.6,-4.89858719658942E-17,0.7));
#11485=CARTESIAN_POINT('Origin',(10.,0.,0.7));
#11486=CARTESIAN_POINT('',(9.6,-4.89858719658942E-17,0.));
#11487=CARTESIAN_POINT('Origin',(2.,0.,0.));
#11488=CARTESIAN_POINT('',(1.6,-4.89858719658941E-17,0.7));
#11489=CARTESIAN_POINT('Origin',(2.,0.,0.7));
#11490=CARTESIAN_POINT('',(1.6,-4.89858719658941E-17,0.));
#11491=CARTESIAN_POINT('Origin',(11.4,-1.53779953703704,0.));
#11492=CARTESIAN_POINT('',(11.4,-1.4227102204299,0.605660349289938));
#11493=CARTESIAN_POINT('Ctrl Pts',(11.4,-1.45718524058191,0.));
#11494=CARTESIAN_POINT('Ctrl Pts',(11.4,-1.45144762186897,0.100853500740053));
#11495=CARTESIAN_POINT('Ctrl Pts',(11.4,-1.44570843451869,0.201707502489292));
#11496=CARTESIAN_POINT('Ctrl Pts',(11.4,-1.43421679834229,0.403593890565801));
#11497=CARTESIAN_POINT('Ctrl Pts',(11.4,-1.42846427656079,0.504627461196798));
#11498=CARTESIAN_POINT('Ctrl Pts',(11.4,-1.4227102204299,0.605660349289938));
#11499=CARTESIAN_POINT('',(11.4,1.4227102204299,0.605660349289938));
#11500=CARTESIAN_POINT('Ctrl Pts',(11.4,1.4227102204299,0.605660349289938));
#11501=CARTESIAN_POINT('Ctrl Pts',(11.4,1.42846501637408,0.504614471147338));
#11502=CARTESIAN_POINT('Ctrl Pts',(11.4,1.43421827757761,0.403567910233218));
#11503=CARTESIAN_POINT('Ctrl Pts',(11.4,1.44570991295315,0.201681522149997));
#11504=CARTESIAN_POINT('Ctrl Pts',(11.4,1.45144836088146,0.100840510682596));
#11505=CARTESIAN_POINT('Ctrl Pts',(11.4,1.45718524058191,0.));
#11506=CARTESIAN_POINT('',(11.4,1.32241589772268,0.7));
#11507=CARTESIAN_POINT('Ctrl Pts',(11.3999999999682,1.32241589773435,0.7));
#11508=CARTESIAN_POINT('Ctrl Pts',(11.4000000023735,1.33035873561384,0.69999999792071));
#11509=CARTESIAN_POINT('Ctrl Pts',(11.3999980827719,1.33823923135401,0.699006238562837));
#11510=CARTESIAN_POINT('Ctrl Pts',(11.3999964146773,1.34591623266897,0.697118452648154));
#11511=CARTESIAN_POINT('Ctrl Pts',(11.3999954805754,1.35021521026861,0.696061327733467));
#11512=CARTESIAN_POINT('Ctrl Pts',(11.3999946303028,1.35445042327231,0.694722827332644));
#11513=CARTESIAN_POINT('Ctrl Pts',(11.3999940855437,1.35859537550353,0.6931136259882));
#11514=CARTESIAN_POINT('Ctrl Pts',(11.3999931076272,1.36603612757745,0.690224891070856));
#11515=CARTESIAN_POINT('Ctrl Pts',(11.3999932937992,1.3731074395729,0.686497549823264));
#11516=CARTESIAN_POINT('Ctrl Pts',(11.3999945206258,1.37966241828116,0.682010734965951));
#11517=CARTESIAN_POINT('Ctrl Pts',(11.3999951957832,1.38326980879772,0.679541513617388));
#11518=CARTESIAN_POINT('Ctrl Pts',(11.399996159718,1.38672054258633,0.67684140394947));
#11519=CARTESIAN_POINT('Ctrl Pts',(11.3999970106794,1.38998612808193,0.67391813047908));
#11520=CARTESIAN_POINT('Ctrl Pts',(11.399997834674,1.39314822810011,0.671087494715186));
#11521=CARTESIAN_POINT('Ctrl Pts',(11.3999985616145,1.39611771109305,0.668064564866167));
#11522=CARTESIAN_POINT('Ctrl Pts',(11.3999985600482,1.39887227052748,0.664860274403491));
#11523=CARTESIAN_POINT('Ctrl Pts',(11.3999985571253,1.40401282028653,0.65888043807832));
#11524=CARTESIAN_POINT('Ctrl Pts',(11.3999962993541,1.40840780441339,0.652270325570232));
#11525=CARTESIAN_POINT('Ctrl Pts',(11.399995545677,1.411994629421,0.6451936465425));
#11526=CARTESIAN_POINT('Ctrl Pts',(11.3999954685939,1.41236147527551,0.644469872631166));
#11527=CARTESIAN_POINT('Ctrl Pts',(11.3999954033687,1.41271982702329,0.643741199273148));
#11528=CARTESIAN_POINT('Ctrl Pts',(11.399995351278,1.41306958904162,0.643007791034547));
#11529=CARTESIAN_POINT('Ctrl Pts',(11.3999948427782,1.41648390439843,0.635848388696429));
#11530=CARTESIAN_POINT('Ctrl Pts',(11.3999960181446,1.41904356023948,0.628323447569199));
#11531=CARTESIAN_POINT('Ctrl Pts',(11.3999977140636,1.42069349507095,0.620600117586001));
#11532=CARTESIAN_POINT('Ctrl Pts',(11.3999987928026,1.4217429844709,0.615687467222433));
#11533=CARTESIAN_POINT('Ctrl Pts',(11.4,1.42242354791745,0.610693903223035));
#11534=CARTESIAN_POINT('Ctrl Pts',(11.4,1.42271022042989,0.605660349289938));
#11535=CARTESIAN_POINT('',(11.4,-1.32241589772233,0.7));
#11536=CARTESIAN_POINT('',(11.4,-0.768899768518519,0.7));
#11537=CARTESIAN_POINT('Ctrl Pts',(11.4,-1.4227102204299,0.605660349289938));
#11538=CARTESIAN_POINT('Ctrl Pts',(11.4,-1.42225988230954,0.613567634148305));
#11539=CARTESIAN_POINT('Ctrl Pts',(11.399997277834,-1.42084002197897,0.621378952482038));
#11540=CARTESIAN_POINT('Ctrl Pts',(11.3999960666067,-1.41853584574224,0.62893480307212));
#11541=CARTESIAN_POINT('Ctrl Pts',(11.3999954054252,-1.41727804822547,0.633059370437125));
#11542=CARTESIAN_POINT('Ctrl Pts',(11.399995101512,-1.41575577202439,0.637107840337094));
#11543=CARTESIAN_POINT('Ctrl Pts',(11.3999952458732,-1.4139766528271,0.641052464558972));
#11544=CARTESIAN_POINT('Ctrl Pts',(11.3999955106959,-1.41071295596475,0.648288661951321));
#11545=CARTESIAN_POINT('Ctrl Pts',(11.3999975070228,-1.40662392062869,0.655096264526915));
#11546=CARTESIAN_POINT('Ctrl Pts',(11.3999983091255,-1.40177626405188,0.661313589686923));
#11547=CARTESIAN_POINT('Ctrl Pts',(11.3999984645713,-1.40083679843637,0.66251849418371));
#11548=CARTESIAN_POINT('Ctrl Pts',(11.3999985618942,-1.3998687022723,0.663701157110503));
#11549=CARTESIAN_POINT('Ctrl Pts',(11.3999985615247,-1.39887227038638,0.664860274403572));
#11550=CARTESIAN_POINT('Ctrl Pts',(11.3999985608543,-1.39706426040285,0.666963474499402));
#11551=CARTESIAN_POINT('Ctrl Pts',(11.3999982409398,-1.39516298427334,0.668989190735049));
#11552=CARTESIAN_POINT('Ctrl Pts',(11.3999977953094,-1.39317470503404,0.670934323115149));
#11553=CARTESIAN_POINT('Ctrl Pts',(11.3999965209597,-1.38748891009577,0.67649673287249));
#11554=CARTESIAN_POINT('Ctrl Pts',(11.3999944455422,-1.38115857071774,0.681340422576046));
#11555=CARTESIAN_POINT('Ctrl Pts',(11.3999937508435,-1.37434881732181,0.685413525744465));
#11556=CARTESIAN_POINT('Ctrl Pts',(11.3999933041982,-1.36997059693002,0.688032261301096));
#11557=CARTESIAN_POINT('Ctrl Pts',(11.3999933336943,-1.3653932120823,0.69033179581025));
#11558=CARTESIAN_POINT('Ctrl Pts',(11.399993839827,-1.36065445462682,0.69228884175444));
#11559=CARTESIAN_POINT('Ctrl Pts',(11.3999946245508,-1.35330733883187,0.695323106179894));
#11560=CARTESIAN_POINT('Ctrl Pts',(11.3999965692242,-1.34565642326237,0.69750197024776));
#11561=CARTESIAN_POINT('Ctrl Pts',(11.3999981510416,-1.33784990929195,0.698756936804364));
#11562=CARTESIAN_POINT('Ctrl Pts',(11.399999182603,-1.33275899381189,0.699575346749464));
#11563=CARTESIAN_POINT('Ctrl Pts',(11.4000000015384,-1.32760128986121,0.699999998642559));
#11564=CARTESIAN_POINT('Ctrl Pts',(11.3999999999682,-1.32241589773435,0.7));
#11565=CARTESIAN_POINT('Ctrl Pts',(11.227882892666,-1.47337141465794,-0.000640335460849732));
#11566=CARTESIAN_POINT('Ctrl Pts',(11.218588765022,-1.46278323638644,0.201451598614313));
#11567=CARTESIAN_POINT('Ctrl Pts',(11.2092944683555,-1.45219508216535,0.40354352620373));
#11568=CARTESIAN_POINT('Ctrl Pts',(11.2000000000001,-1.44160695250309,0.60563544721184));
#11569=CARTESIAN_POINT('Ctrl Pts',(10.1843397214697,-1.57034855377304,-0.000384310983874139));
#11570=CARTESIAN_POINT('Ctrl Pts',(10.1768953195658,-1.55975965902304,0.201708049868595));
#11571=CARTESIAN_POINT('Ctrl Pts',(10.1694507716805,-1.54917076711515,0.403800406245857));
#11572=CARTESIAN_POINT('Ctrl Pts',(10.1620060668616,-1.53858190981164,0.605892758286982));
#11573=CARTESIAN_POINT('Ctrl Pts',(9.14170648965309,-1.65016851777514,-0.000148134864058495));
#11574=CARTESIAN_POINT('Ctrl Pts',(9.13611341817177,-1.63957870617509,0.201944615677573));
#11575=CARTESIAN_POINT('Ctrl Pts',(9.13052023035058,-1.6289888900612,0.404037363603497));
#11576=CARTESIAN_POINT('Ctrl Pts',(9.124926910836,-1.6183991014662,0.606130109186173));
#11577=CARTESIAN_POINT('Ctrl Pts',(8.1,-1.69866351109718,1.00613961606655E-16));
#11578=CARTESIAN_POINT('Ctrl Pts',(8.09625995443094,-1.68807302815665,0.202092993803311));
#11579=CARTESIAN_POINT('Ctrl Pts',(8.09251982249141,-1.67748255132318,0.404185986335255));
#11580=CARTESIAN_POINT('Ctrl Pts',(8.08877960280056,-1.66689208072706,0.606278977577217));
#11581=CARTESIAN_POINT('Ctrl Pts',(8.1,-1.66641703131627,0.605314487869832));
#11582=CARTESIAN_POINT('Ctrl Pts',(9.13548525483003,-1.617718421277,0.605389190939432));
#11583=CARTESIAN_POINT('Ctrl Pts',(10.168822041161,-1.53796707615457,0.605507632815633));
#11584=CARTESIAN_POINT('Ctrl Pts',(11.2000000000893,-1.44160695345912,0.605635447210802));
#11585=CARTESIAN_POINT('Ctrl Pts',(11.7095939787209,-1.42740645209206,-7.69249563980189E-5));
#11586=CARTESIAN_POINT('Ctrl Pts',(11.6994545874061,-1.41682738380082,0.201847033339061));
#11587=CARTESIAN_POINT('Ctrl Pts',(11.6893150192885,-1.40624834198077,0.403770984173611));
#11588=CARTESIAN_POINT('Ctrl Pts',(11.6791752715866,-1.39566932719028,0.605694927437301));
#11589=CARTESIAN_POINT('Ctrl Pts',(11.6063871276792,-1.43748358609578,-5.11721697277706E-5));
#11590=CARTESIAN_POINT('Ctrl Pts',(11.596430427176,-1.42690445239132,0.201872829148883));
#11591=CARTESIAN_POINT('Ctrl Pts',(11.5864735514701,-1.41632534465399,0.403796823219986));
#11592=CARTESIAN_POINT('Ctrl Pts',(11.5765164978042,-1.40574626343445,0.605720809936841));
#11593=CARTESIAN_POINT('Ctrl Pts',(11.5031891278894,-1.4474144288224,-2.55082377288765E-5));
#11594=CARTESIAN_POINT('Ctrl Pts',(11.4934151336386,-1.43683522760458,0.201898535909597));
#11595=CARTESIAN_POINT('Ctrl Pts',(11.4836409658656,-1.42625605183456,0.40382257302165));
#11596=CARTESIAN_POINT('Ctrl Pts',(11.4738666218385,-1.41567690205216,0.605746602994839));
#11597=CARTESIAN_POINT('Ctrl Pts',(11.4,-1.45718524058191,-5.20417042793042E-18));
#11598=CARTESIAN_POINT('Ctrl Pts',(11.3904087275488,-1.44660597001679,0.201924086674796));
#11599=CARTESIAN_POINT('Ctrl Pts',(11.3808172833376,-1.43602672436683,0.403848166524883));
#11600=CARTESIAN_POINT('Ctrl Pts',(11.3712256646606,-1.42544750415802,0.605772239449758));
#11601=CARTESIAN_POINT('',(11.6778970386953,-1.39579479040469,0.605695249702977));
#11602=CARTESIAN_POINT('Ctrl Pts',(11.4,-1.4227102204299,0.605660349289938));
#11603=CARTESIAN_POINT('Ctrl Pts',(11.4926474653491,-1.41386220753305,0.605671932550561));
#11604=CARTESIAN_POINT('Ctrl Pts',(11.585279512325,-1.40488700096013,0.605683574233495));
#11605=CARTESIAN_POINT('Ctrl Pts',(11.6778970386953,-1.39579479040469,0.605695249702977));
#11606=CARTESIAN_POINT('Ctrl Pts',(11.6778970386953,-1.39579479040469,0.605695249702977));
#11607=CARTESIAN_POINT('Ctrl Pts',(11.6884613130147,-1.40633044792991,0.403796817797553));
#11608=CARTESIAN_POINT('Ctrl Pts',(11.6990256725537,-1.41686632615463,0.201898401304098));
#11609=CARTESIAN_POINT('Ctrl Pts',(11.7095901160181,-1.42740242188993,5.19332840620557E-17));
#11610=CARTESIAN_POINT('Ctrl Pts',(11.2,-1.34133050917871,0.7));
#11611=CARTESIAN_POINT('Ctrl Pts',(10.1668086441106,-1.43797263608903,0.7));
#11612=CARTESIAN_POINT('Ctrl Pts',(9.13190264019122,-1.51792184128158,0.7));
#11613=CARTESIAN_POINT('Ctrl Pts',(8.09530923905977,-1.56666858280461,0.7));
#11614=CARTESIAN_POINT('Ctrl Pts',(11.2026864299662,-1.37005086445236,0.7));
#11615=CARTESIAN_POINT('Ctrl Pts',(10.1691860218014,-1.46674693471719,0.700000910790016));
#11616=CARTESIAN_POINT('Ctrl Pts',(9.13384227773975,-1.54675516497,0.699999464833944));
#11617=CARTESIAN_POINT('Ctrl Pts',(8.09666712422266,-1.59554384206015,0.700000000000001));
#11618=CARTESIAN_POINT('Ctrl Pts',(11.2073428085028,-1.4198317437391,0.676744232988519));
#11619=CARTESIAN_POINT('Ctrl Pts',(10.1733099382853,-1.51661799675652,0.676702307311825));
#11620=CARTESIAN_POINT('Ctrl Pts',(9.13719745543551,-1.59672983278297,0.676663906627884));
#11621=CARTESIAN_POINT('Ctrl Pts',(8.09902054834098,-1.64558911349573,0.676639354455264));
#11622=CARTESIAN_POINT('Ctrl Pts',(11.2091847227485,-1.43952346553595,0.627236497176141));
#11623=CARTESIAN_POINT('Ctrl Pts',(10.1749352046592,-1.53629892039422,0.62712791425818));
#11624=CARTESIAN_POINT('Ctrl Pts',(9.13852107143019,-1.61640633519008,0.627027713743691));
#11625=CARTESIAN_POINT('Ctrl Pts',(8.0999458765183,-1.66526610220338,0.626964226563296));
#11626=CARTESIAN_POINT('Ctrl Pts',(11.209298290232,-1.4407376041935,0.605636599993194));
#11627=CARTESIAN_POINT('Ctrl Pts',(10.1750338985877,-1.53748737250229,0.605508345221004));
#11628=CARTESIAN_POINT('Ctrl Pts',(9.13859765097935,-1.61757204607208,0.605389415477198));
#11629=CARTESIAN_POINT('Ctrl Pts',(8.1,-1.66641703131627,0.605314487869832));
#11630=CARTESIAN_POINT('Ctrl Pts',(11.2,-1.34133050917871,0.7));
#11631=CARTESIAN_POINT('Ctrl Pts',(10.16836710286,-1.43782686176815,0.7));
#11632=CARTESIAN_POINT('Ctrl Pts',(9.13502472651537,-1.51768061363633,0.7));
#11633=CARTESIAN_POINT('Ctrl Pts',(8.09999999865516,-1.56644778212326,0.7));
#11634=CARTESIAN_POINT('Ctrl Pts',(11.6681436286308,-1.2964346619681,0.7));
#11635=CARTESIAN_POINT('Ctrl Pts',(11.5756099286391,-1.3055179747114,0.7));
#11636=CARTESIAN_POINT('Ctrl Pts',(11.4830653488871,-1.31448403714215,0.7));
#11637=CARTESIAN_POINT('Ctrl Pts',(11.3905090053564,-1.32332268868375,0.7));
#11638=CARTESIAN_POINT('Ctrl Pts',(11.6709605510772,-1.32513126902304,0.700000000000001));
#11639=CARTESIAN_POINT('Ctrl Pts',(11.5784027531871,-1.33421922733773,0.700000082825348));
#11640=CARTESIAN_POINT('Ctrl Pts',(11.4858332859074,-1.34318985044544,0.699999917777441));
#11641=CARTESIAN_POINT('Ctrl Pts',(11.3932507170007,-1.35203326785046,0.7));
#11642=CARTESIAN_POINT('Ctrl Pts',(11.6758431636759,-1.37487151491717,0.67676311428296));
#11643=CARTESIAN_POINT('Ctrl Pts',(11.583243842395,-1.38396722707511,0.676759299309384));
#11644=CARTESIAN_POINT('Ctrl Pts',(11.4906306781253,-1.39294591144353,0.676755553516685));
#11645=CARTESIAN_POINT('Ctrl Pts',(11.3980029235659,-1.40179729139028,0.67675176769038));
#11646=CARTESIAN_POINT('Ctrl Pts',(11.6777767156198,-1.39456903283364,0.627286048421068));
#11647=CARTESIAN_POINT('Ctrl Pts',(11.5851604051362,-1.40366358810601,0.627276165220861));
#11648=CARTESIAN_POINT('Ctrl Pts',(11.4925297866457,-1.41264104586547,0.627266369072496));
#11649=CARTESIAN_POINT('Ctrl Pts',(11.3998836071583,-1.4214913811319,0.627256563056779));
#11650=CARTESIAN_POINT('Ctrl Pts',(11.6778970386953,-1.39579479040469,0.605695249702977));
#11651=CARTESIAN_POINT('Ctrl Pts',(11.585279512325,-1.40488700096013,0.605683574233495));
#11652=CARTESIAN_POINT('Ctrl Pts',(11.4926474653491,-1.41386220753305,0.605671932550561));
#11653=CARTESIAN_POINT('Ctrl Pts',(11.4,-1.4227102204299,0.605660349289938));
#11654=CARTESIAN_POINT('',(11.6681436286308,-1.2964346619681,0.7));
#11655=CARTESIAN_POINT('Ctrl Pts',(11.6681436286308,-1.2964346619681,0.7));
#11656=CARTESIAN_POINT('Ctrl Pts',(11.5787728332608,-1.30520749699507,0.7));
#11657=CARTESIAN_POINT('Ctrl Pts',(11.4893918891838,-1.31387096021207,0.7));
#11658=CARTESIAN_POINT('Ctrl Pts',(11.3999999999682,-1.32241589773435,0.7));
#11659=CARTESIAN_POINT('Origin',(11.6681436286308,-1.2964346619681,0.6));
#11660=CARTESIAN_POINT('Origin',(6.08012166120517,1.06778195214465E-16,
0.7));
#11661=CARTESIAN_POINT('Ctrl Pts',(8.0999999986552,1.56644778212326,0.7));
#11662=CARTESIAN_POINT('Ctrl Pts',(9.13502472651542,1.51768061363633,0.7));
#11663=CARTESIAN_POINT('Ctrl Pts',(10.16836710286,1.43782686176815,0.7));
#11664=CARTESIAN_POINT('Ctrl Pts',(11.2,1.34133050917871,0.7));
#11665=CARTESIAN_POINT('Origin',(6.08012166120517,1.06778195214465E-16,
0.7));
#11666=CARTESIAN_POINT('',(11.6681436286308,1.2964346619681,0.7));
#11667=CARTESIAN_POINT('Ctrl Pts',(11.3999999999682,1.32241589773435,0.7));
#11668=CARTESIAN_POINT('Ctrl Pts',(11.4893918891837,1.31387096021208,0.7));
#11669=CARTESIAN_POINT('Ctrl Pts',(11.5787728332608,1.30520749699508,0.7));
#11670=CARTESIAN_POINT('Ctrl Pts',(11.6681436286308,1.2964346619681,0.7));
#11671=CARTESIAN_POINT('',(11.6681436286308,0.8,0.7));
#11672=CARTESIAN_POINT('Ctrl Pts',(8.09530923905978,1.56666858280461,0.7));
#11673=CARTESIAN_POINT('Ctrl Pts',(9.13190264019124,1.51792184128158,0.7));
#11674=CARTESIAN_POINT('Ctrl Pts',(10.1668086441106,1.43797263608903,0.7));
#11675=CARTESIAN_POINT('Ctrl Pts',(11.2,1.34133050917871,0.7));
#11676=CARTESIAN_POINT('Ctrl Pts',(8.09666712422266,1.59554384206015,0.700000000000001));
#11677=CARTESIAN_POINT('Ctrl Pts',(9.13384227773977,1.54675516497,0.699999464833944));
#11678=CARTESIAN_POINT('Ctrl Pts',(10.1691860218013,1.46674693471719,0.700000910790016));
#11679=CARTESIAN_POINT('Ctrl Pts',(11.2026864299662,1.37005086445236,0.7));
#11680=CARTESIAN_POINT('Ctrl Pts',(8.09902054834099,1.64558911349573,0.676639354455264));
#11681=CARTESIAN_POINT('Ctrl Pts',(9.13719745543553,1.59672983278297,0.676663906627884));
#11682=CARTESIAN_POINT('Ctrl Pts',(10.1733099382853,1.51661799675652,0.676702307311825));
#11683=CARTESIAN_POINT('Ctrl Pts',(11.2073428085028,1.4198317437391,0.676744232988519));
#11684=CARTESIAN_POINT('Ctrl Pts',(8.0999458765183,1.66526610220338,0.626964226563296));
#11685=CARTESIAN_POINT('Ctrl Pts',(9.1385210714302,1.61640633519008,0.627027713743691));
#11686=CARTESIAN_POINT('Ctrl Pts',(10.1749352046592,1.53629892039423,0.62712791425818));
#11687=CARTESIAN_POINT('Ctrl Pts',(11.2091847227485,1.43952346553595,0.627236497176141));
#11688=CARTESIAN_POINT('Ctrl Pts',(8.1,1.66641703131627,0.605314487869832));
#11689=CARTESIAN_POINT('Ctrl Pts',(9.13859765097937,1.61757204607208,0.605389415477198));
#11690=CARTESIAN_POINT('Ctrl Pts',(10.1750338985877,1.53748737250229,0.605508345221004));
#11691=CARTESIAN_POINT('Ctrl Pts',(11.209298290232,1.4407376041935,0.605636599993194));
#11692=CARTESIAN_POINT('Ctrl Pts',(11.2000000000893,1.44160695345912,0.605635447210802));
#11693=CARTESIAN_POINT('Ctrl Pts',(10.168822041161,1.53796707615457,0.605507632815633));
#11694=CARTESIAN_POINT('Ctrl Pts',(9.13548525483005,1.617718421277,0.605389190939432));
#11695=CARTESIAN_POINT('Ctrl Pts',(8.1,1.66641703131627,0.605314487869832));
#11696=CARTESIAN_POINT('Ctrl Pts',(8.1,1.69866351109859,-2.6441702993818E-11));
#11697=CARTESIAN_POINT('Ctrl Pts',(8.09625995443078,1.68807302815759,0.202092993785684));
#11698=CARTESIAN_POINT('Ctrl Pts',(8.09251982249108,1.67748255132366,0.404185986326441));
#11699=CARTESIAN_POINT('Ctrl Pts',(8.08877960280008,1.66689208072708,0.606278977577217));
#11700=CARTESIAN_POINT('Ctrl Pts',(9.14170648965349,1.65016851777655,-0.00014813489050026));
#11701=CARTESIAN_POINT('Ctrl Pts',(9.13611341817193,1.63957870617604,0.201944615659945));
#11702=CARTESIAN_POINT('Ctrl Pts',(9.1305202303505,1.62898889006169,0.404037363594684));
#11703=CARTESIAN_POINT('Ctrl Pts',(9.12492691083567,1.61839910146622,0.606130109186173));
#11704=CARTESIAN_POINT('Ctrl Pts',(10.1843397214705,1.57034855377444,-0.000384311010315772));
#11705=CARTESIAN_POINT('Ctrl Pts',(10.1768953195662,1.55975965902398,0.201708049850968));
#11706=CARTESIAN_POINT('Ctrl Pts',(10.1694507716807,1.54917076711562,0.403800406237042));
#11707=CARTESIAN_POINT('Ctrl Pts',(10.1620060668615,1.53858190981166,0.605892758286982));
#11708=CARTESIAN_POINT('Ctrl Pts',(11.2278828926672,1.47337141465933,-0.000640335487291374));
#11709=CARTESIAN_POINT('Ctrl Pts',(11.2185887650228,1.46278323638736,0.201451598596686));
#11710=CARTESIAN_POINT('Ctrl Pts',(11.2092944683559,1.45219508216582,0.403543526194916));
#11711=CARTESIAN_POINT('Ctrl Pts',(11.2000000000001,1.44160695250309,0.60563544721184));
#11712=CARTESIAN_POINT('Ctrl Pts',(11.4,1.45718524058191,-1.37043154602168E-16));
#11713=CARTESIAN_POINT('Ctrl Pts',(11.3904087275488,1.44660597001679,0.201924086674796));
#11714=CARTESIAN_POINT('Ctrl Pts',(11.3808172833376,1.43602672436683,0.403848166524884));
#11715=CARTESIAN_POINT('Ctrl Pts',(11.3712256646606,1.42544750415802,0.605772239449759));
#11716=CARTESIAN_POINT('Ctrl Pts',(11.5031891278894,1.4474144288224,-2.55082377290153E-5));
#11717=CARTESIAN_POINT('Ctrl Pts',(11.4934151336386,1.43683522760458,0.201898535909598));
#11718=CARTESIAN_POINT('Ctrl Pts',(11.4836409658656,1.42625605183455,0.40382257302165));
#11719=CARTESIAN_POINT('Ctrl Pts',(11.4738666218385,1.41567690205216,0.605746602994839));
#11720=CARTESIAN_POINT('Ctrl Pts',(11.6063871276792,1.43748358609579,-5.1172169727805E-5));
#11721=CARTESIAN_POINT('Ctrl Pts',(11.596430427176,1.42690445239132,0.201872829148883));
#11722=CARTESIAN_POINT('Ctrl Pts',(11.5864735514701,1.41632534465399,0.403796823219986));
#11723=CARTESIAN_POINT('Ctrl Pts',(11.5765164978042,1.40574626343445,0.605720809936842));
#11724=CARTESIAN_POINT('Ctrl Pts',(11.7095939787209,1.42740645209206,-7.69249563980588E-5));
#11725=CARTESIAN_POINT('Ctrl Pts',(11.6994545874061,1.41682738380082,0.201847033339061));
#11726=CARTESIAN_POINT('Ctrl Pts',(11.6893150192885,1.40624834198077,0.403770984173611));
#11727=CARTESIAN_POINT('Ctrl Pts',(11.6791752715866,1.39566932719028,0.605694927437301));
#11728=CARTESIAN_POINT('',(11.6778970386953,1.39579479040469,0.605695249702977));
#11729=CARTESIAN_POINT('Ctrl Pts',(11.7095901160181,1.42740242188993,2.01986864734049E-16));
#11730=CARTESIAN_POINT('Ctrl Pts',(11.6990256725537,1.41686632615463,0.201898401304098));
#11731=CARTESIAN_POINT('Ctrl Pts',(11.6884613130147,1.40633044792991,0.403796817797553));
#11732=CARTESIAN_POINT('Ctrl Pts',(11.6778970386953,1.39579479040469,0.605695249702978));
#11733=CARTESIAN_POINT('Ctrl Pts',(11.6778970386953,1.39579479040469,0.605695249702977));
#11734=CARTESIAN_POINT('Ctrl Pts',(11.585279512325,1.40488700096013,0.605683574233495));
#11735=CARTESIAN_POINT('Ctrl Pts',(11.4926474653491,1.41386220753305,0.605671932550561));
#11736=CARTESIAN_POINT('Ctrl Pts',(11.4,1.4227102204299,0.605660349289938));
#11737=CARTESIAN_POINT('Origin',(7.9,1.7737037037037,0.));
#11738=CARTESIAN_POINT('',(7.9,-1.67543132363858,0.605300614462415));
#11739=CARTESIAN_POINT('Ctrl Pts',(7.9,-1.67543132363858,0.605300614462415));
#11740=CARTESIAN_POINT('Ctrl Pts',(7.9,-1.68078196203297,0.504592238472094));
#11741=CARTESIAN_POINT('Ctrl Pts',(7.9,-1.68613236521525,0.403883028813119));
#11742=CARTESIAN_POINT('Ctrl Pts',(7.9,-1.69685110017509,0.202116711316755));
#11743=CARTESIAN_POINT('Ctrl Pts',(7.9,-1.70221951791351,0.10105794916591));
#11744=CARTESIAN_POINT('Ctrl Pts',(7.9,-1.70758761671949,0.));
#11745=CARTESIAN_POINT('',(7.9,-1.57547905376932,0.7));
#11746=CARTESIAN_POINT('Ctrl Pts',(7.9,-1.57547905376882,0.7));
#11747=CARTESIAN_POINT('Ctrl Pts',(7.9,-1.58339333479856,0.700000000000001));
#11748=CARTESIAN_POINT('Ctrl Pts',(7.89999913038498,-1.59124411312484,0.699006032637452));
#11749=CARTESIAN_POINT('Ctrl Pts',(7.89999837104309,-1.59889106951376,0.697118831203047));
#11750=CARTESIAN_POINT('Ctrl Pts',(7.89999794343345,-1.6031973145812,0.696056087876834));
#11751=CARTESIAN_POINT('Ctrl Pts',(7.89999755365678,-1.60743898057435,0.694709047589066));
#11752=CARTESIAN_POINT('Ctrl Pts',(7.89999730661842,-1.61158931211603,0.693088720937666));
#11753=CARTESIAN_POINT('Ctrl Pts',(7.89999686465941,-1.6190143793929,0.690189908089508));
#11754=CARTESIAN_POINT('Ctrl Pts',(7.89999696143539,-1.626066934352,0.686450944759811));
#11755=CARTESIAN_POINT('Ctrl Pts',(7.89999752554231,-1.63260082031789,0.681953255064161));
#11756=CARTESIAN_POINT('Ctrl Pts',(7.89999783650325,-1.63620259020663,0.679473927540052));
#11757=CARTESIAN_POINT('Ctrl Pts',(7.89999827825103,-1.63964648551863,0.676763160200805));
#11758=CARTESIAN_POINT('Ctrl Pts',(7.89999867021687,-1.64290407802379,0.673829034208746));
#11759=CARTESIAN_POINT('Ctrl Pts',(7.89999905115172,-1.64606999298761,0.670977482527793));
#11760=CARTESIAN_POINT('Ctrl Pts',(7.89999938859403,-1.64904076201529,0.667932171841817));
#11761=CARTESIAN_POINT('Ctrl Pts',(7.89999938783828,-1.6517939440564,0.66470449824639));
#11762=CARTESIAN_POINT('Ctrl Pts',(7.89999938643498,-1.65690611124346,0.658711285012161));
#11763=CARTESIAN_POINT('Ctrl Pts',(7.89999834643869,-1.661271022418,0.652090721578155));
#11764=CARTESIAN_POINT('Ctrl Pts',(7.89999799057748,-1.66482884904143,0.645008203309728));
#11765=CARTESIAN_POINT('Ctrl Pts',(7.89999795399159,-1.66519462718329,0.644280053614395));
#11766=CARTESIAN_POINT('Ctrl Pts',(7.89999792287445,-1.66555183396469,0.643547001244109));
#11767=CARTESIAN_POINT('Ctrl Pts',(7.89999789784292,-1.66590037542058,0.642809214685104));
#11768=CARTESIAN_POINT('Ctrl Pts',(7.89999765441981,-1.66928982250308,0.635634491398386));
#11769=CARTESIAN_POINT('Ctrl Pts',(7.89999817709027,-1.67182454272713,0.628096763436417));
#11770=CARTESIAN_POINT('Ctrl Pts',(7.8999989464625,-1.67345106343068,0.620364350320046));
#11771=CARTESIAN_POINT('Ctrl Pts',(7.89999943944948,-1.67449328136075,0.615409688768565));
#11772=CARTESIAN_POINT('Ctrl Pts',(7.89999999630063,-1.67516175160204,0.610374426093907));
#11773=CARTESIAN_POINT('Ctrl Pts',(7.89999999769359,-1.67543132314592,0.605300614465834));
#11774=CARTESIAN_POINT('',(7.9,1.57547905376882,0.7));
#11775=CARTESIAN_POINT('',(7.9,0.886851851851852,0.7));
#11776=CARTESIAN_POINT('',(7.9,1.67543132363858,0.605300614462415));
#11777=CARTESIAN_POINT('Ctrl Pts',(7.89999999769359,1.67543132314592,0.605300614465834));
#11778=CARTESIAN_POINT('Ctrl Pts',(7.89999999552123,1.67501091691767,0.613213400729193));
#11779=CARTESIAN_POINT('Ctrl Pts',(7.89999875799714,1.67362284400845,0.621034919585595));
#11780=CARTESIAN_POINT('Ctrl Pts',(7.89999821041927,1.67135120200026,0.628604813990272));
#11781=CARTESIAN_POINT('Ctrl Pts',(7.89999790518813,1.67008494211401,0.632824428521627));
#11782=CARTESIAN_POINT('Ctrl Pts',(7.89999777089825,1.66854314417455,0.636965893954691));
#11783=CARTESIAN_POINT('Ctrl Pts',(7.89999784944871,1.66673368022774,0.640999456224326));
#11784=CARTESIAN_POINT('Ctrl Pts',(7.89999799035603,1.66348778281681,0.648235040746992));
#11785=CARTESIAN_POINT('Ctrl Pts',(7.8999989183875,1.65941887886545,0.655045206964536));
#11786=CARTESIAN_POINT('Ctrl Pts',(7.89999927807636,1.65459101651367,0.661266862646797));
#11787=CARTESIAN_POINT('Ctrl Pts',(7.89999934554656,1.65368540929837,0.662433916689859));
#11788=CARTESIAN_POINT('Ctrl Pts',(7.89999938740919,1.65275296801062,0.663580193269421));
#11789=CARTESIAN_POINT('Ctrl Pts',(7.89999938728957,1.65179394408007,0.664704498246374));
#11790=CARTESIAN_POINT('Ctrl Pts',(7.89999938705343,1.64990069294102,0.666924037937161));
#11791=CARTESIAN_POINT('Ctrl Pts',(7.89999922461202,1.64790387543569,0.669057997255949));
#11792=CARTESIAN_POINT('Ctrl Pts',(7.89999900301747,1.64581073954063,0.671102663899023));
#11793=CARTESIAN_POINT('Ctrl Pts',(7.89999840121276,1.64012621790684,0.676655553128015));
#11794=CARTESIAN_POINT('Ctrl Pts',(7.89999746538644,1.63379824275617,0.681490110487894));
#11795=CARTESIAN_POINT('Ctrl Pts',(7.89999715581736,1.6269906793715,0.685552192443336));
#11796=CARTESIAN_POINT('Ctrl Pts',(7.89999695885968,1.62265949106942,0.688136618155352));
#11797=CARTESIAN_POINT('Ctrl Pts',(7.89999697413705,1.61813320929371,0.690407672840119));
#11798=CARTESIAN_POINT('Ctrl Pts',(7.89999720528031,1.61344832872307,0.692342105328139));
#11799=CARTESIAN_POINT('Ctrl Pts',(7.89999756646959,1.60612763680413,0.69536488980882));
#11800=CARTESIAN_POINT('Ctrl Pts',(7.89999845750109,1.59850458633822,0.69753330980446));
#11801=CARTESIAN_POINT('Ctrl Pts',(7.89999917312139,1.59072625322659,0.698777780766876));
#11802=CARTESIAN_POINT('Ctrl Pts',(7.8999996358458,1.58569673594883,0.699582463224842));
#11803=CARTESIAN_POINT('Ctrl Pts',(7.9,1.58060170040825,0.7));
#11804=CARTESIAN_POINT('Ctrl Pts',(7.9,1.57547905376882,0.7));
#11805=CARTESIAN_POINT('Ctrl Pts',(7.9,1.70758761671949,0.));
#11806=CARTESIAN_POINT('Ctrl Pts',(7.9,1.70221949782947,0.101058327261027));
#11807=CARTESIAN_POINT('Ctrl Pts',(7.9,1.69685105999395,0.202117467714));
#11808=CARTESIAN_POINT('Ctrl Pts',(7.9,1.68613232500772,0.403883785628764));
#11809=CARTESIAN_POINT('Ctrl Pts',(7.9,1.6807819419292,0.504592616860323));
#11810=CARTESIAN_POINT('Ctrl Pts',(7.9,1.67543132363858,0.605300614462415));
#11811=CARTESIAN_POINT('Ctrl Pts',(7.91019312999368,-1.70715886092982,-0.000134090250286965));
#11812=CARTESIAN_POINT('Ctrl Pts',(7.90679525219671,-1.69658223918655,0.201692187253877));
#11813=CARTESIAN_POINT('Ctrl Pts',(7.90339729501941,-1.68600562260833,0.40351846369823));
#11814=CARTESIAN_POINT('Ctrl Pts',(7.89999925719352,-1.67542901130525,0.605344739067286));
#11815=CARTESIAN_POINT('Ctrl Pts',(6.63535348802246,-1.76179300886274,3.38453142643293E-5));
#11816=CARTESIAN_POINT('Ctrl Pts',(6.63422081661327,-1.7512156246026,0.201860399405878));
#11817=CARTESIAN_POINT('Ctrl Pts',(6.6330881724013,-1.74063821514668,0.403686949685767));
#11818=CARTESIAN_POINT('Ctrl Pts',(6.63195543348167,-1.7300608292057,0.605513504373875));
#11819=CARTESIAN_POINT('Ctrl Pts',(5.36191629096386,-1.76821426310706,6.25694230841134E-5));
#11820=CARTESIAN_POINT('Ctrl Pts',(5.36305144950513,-1.75763653444312,0.201889164820622));
#11821=CARTESIAN_POINT('Ctrl Pts',(5.36418670601529,-1.74705878452761,0.403715755186214));
#11822=CARTESIAN_POINT('Ctrl Pts',(5.36532191986746,-1.73648104871457,0.605542351516859));
#11823=CARTESIAN_POINT('Ctrl Pts',(4.08978435919194,-1.70060618495018,-0.000163379468877527));
#11824=CARTESIAN_POINT('Ctrl Pts',(4.09318947412453,-1.69002991101751,0.201662855819258));
#11825=CARTESIAN_POINT('Ctrl Pts',(4.09659468720556,-1.67945364498778,0.403489089874722));
#11826=CARTESIAN_POINT('Ctrl Pts',(4.1,-1.66887738702936,0.605315322680078));
#11827=CARTESIAN_POINT('Ctrl Pts',(4.10000000006189,-1.66887738587128,0.605315322687833));
#11828=CARTESIAN_POINT('Ctrl Pts',(5.36600428635239,-1.73653511802878,0.605201749988751));
#11829=CARTESIAN_POINT('Ctrl Pts',(6.63469107356441,-1.72995836404769,0.605216415547347));
#11830=CARTESIAN_POINT('Ctrl Pts',(7.89999999997453,-1.67543132304763,0.605300614465986));
#11831=CARTESIAN_POINT('Ctrl Pts',(7.9,-1.57547905376882,0.7));
#11832=CARTESIAN_POINT('Ctrl Pts',(6.63400208894818,-1.63014048526579,0.7));
#11833=CARTESIAN_POINT('Ctrl Pts',(5.36531976402288,-1.63670020240541,0.7));
#11834=CARTESIAN_POINT('Ctrl Pts',(4.09999999999999,-1.56887583540973,0.7));
#11835=CARTESIAN_POINT('Ctrl Pts',(7.9012470621039,-1.60436190544783,0.700000000000001));
#11836=CARTESIAN_POINT('Ctrl Pts',(6.6345175325877,-1.65907137725265,0.700000604190856));
#11837=CARTESIAN_POINT('Ctrl Pts',(5.36490325870521,-1.66564852467601,0.700000815814724));
#11838=CARTESIAN_POINT('Ctrl Pts',(4.09845273665223,-1.59774131518914,0.699999999999999));
#11839=CARTESIAN_POINT('Ctrl Pts',(7.90340849276168,-1.6544221878571,0.676636720659303));
#11840=CARTESIAN_POINT('Ctrl Pts',(6.63541917043928,-1.70921256696412,0.676609005714152));
#11841=CARTESIAN_POINT('Ctrl Pts',(5.36416860778507,-1.71581908642683,0.67660414986632));
#11842=CARTESIAN_POINT('Ctrl Pts',(4.09577098158984,-1.64777167791894,0.676641578059328));
#11843=CARTESIAN_POINT('Ctrl Pts',(7.90425799286387,-1.67409721877663,0.626952737571144));
#11844=CARTESIAN_POINT('Ctrl Pts',(6.63576820027036,-1.72888861107585,0.626881076846221));
#11845=CARTESIAN_POINT('Ctrl Pts',(5.36388821219926,-1.73550154452763,0.626868555890157));
#11846=CARTESIAN_POINT('Ctrl Pts',(4.09471668402893,-1.66744047248441,0.626965338598652));
#11847=CARTESIAN_POINT('Ctrl Pts',(7.90430757201307,-1.67524550738887,0.605300901379154));
#11848=CARTESIAN_POINT('Ctrl Pts',(6.63578978311492,-1.73002023206136,0.605216330280387));
#11849=CARTESIAN_POINT('Ctrl Pts',(5.3638700255334,-1.7366305488338,0.605201579557148));
#11850=CARTESIAN_POINT('Ctrl Pts',(4.09465499692593,-1.6685912965035,0.605315802949303));
#11851=CARTESIAN_POINT('Ctrl Pts',(7.9,-1.57547905376882,0.7));
#11852=CARTESIAN_POINT('Ctrl Pts',(6.63400208894818,-1.63014048526579,0.7));
#11853=CARTESIAN_POINT('Ctrl Pts',(5.36531976402288,-1.63670020240541,0.7));
#11854=CARTESIAN_POINT('Ctrl Pts',(4.09999999999999,-1.56887583540973,0.7));
#11855=CARTESIAN_POINT('Origin',(6.08012166120517,1.06778195214465E-16,
0.7));
#11856=CARTESIAN_POINT('Ctrl Pts',(4.1,1.56887583540973,0.7));
#11857=CARTESIAN_POINT('Ctrl Pts',(5.36531976402291,1.63670020240541,0.7));
#11858=CARTESIAN_POINT('Ctrl Pts',(6.63400208894819,1.63014048526579,0.7));
#11859=CARTESIAN_POINT('Ctrl Pts',(7.9,1.57547905376882,0.7));
#11860=CARTESIAN_POINT('Ctrl Pts',(4.1,1.56887583540973,0.7));
#11861=CARTESIAN_POINT('Ctrl Pts',(5.36531976402291,1.63670020240541,0.7));
#11862=CARTESIAN_POINT('Ctrl Pts',(6.63400208894819,1.63014048526579,0.7));
#11863=CARTESIAN_POINT('Ctrl Pts',(7.9,1.57547905376882,0.7));
#11864=CARTESIAN_POINT('Ctrl Pts',(4.09845273665224,1.59774131518914,0.699999999999999));
#11865=CARTESIAN_POINT('Ctrl Pts',(5.36490325870523,1.66564852467601,0.700000815814725));
#11866=CARTESIAN_POINT('Ctrl Pts',(6.6345175325877,1.65907137725265,0.700000604190856));
#11867=CARTESIAN_POINT('Ctrl Pts',(7.9012470621039,1.60436190544783,0.700000000000001));
#11868=CARTESIAN_POINT('Ctrl Pts',(4.09577098158985,1.64777167791894,0.676641578059328));
#11869=CARTESIAN_POINT('Ctrl Pts',(5.36416860778509,1.71581908642683,0.67660414986632));
#11870=CARTESIAN_POINT('Ctrl Pts',(6.6354191704393,1.70921256696412,0.676609005714152));
#11871=CARTESIAN_POINT('Ctrl Pts',(7.90340849276168,1.6544221878571,0.676636720659302));
#11872=CARTESIAN_POINT('Ctrl Pts',(4.09471668402895,1.66744047248441,0.626965338598652));
#11873=CARTESIAN_POINT('Ctrl Pts',(5.36388821219928,1.73550154452763,0.626868555890157));
#11874=CARTESIAN_POINT('Ctrl Pts',(6.63576820027036,1.72888861107585,0.626881076846221));
#11875=CARTESIAN_POINT('Ctrl Pts',(7.90425799286387,1.67409721877663,0.626952737571144));
#11876=CARTESIAN_POINT('Ctrl Pts',(4.09465499692594,1.6685912965035,0.605315802949303));
#11877=CARTESIAN_POINT('Ctrl Pts',(5.36387002553342,1.7366305488338,0.605201579557148));
#11878=CARTESIAN_POINT('Ctrl Pts',(6.63578978311492,1.73002023206136,0.605216330280387));
#11879=CARTESIAN_POINT('Ctrl Pts',(7.90430757201307,1.67524550738887,0.605300901379154));
#11880=CARTESIAN_POINT('Ctrl Pts',(7.89999999997454,1.67543132304763,0.605300614465986));
#11881=CARTESIAN_POINT('Ctrl Pts',(6.63469107356441,1.72995836404769,0.605216415547348));
#11882=CARTESIAN_POINT('Ctrl Pts',(5.36600428635241,1.73653511802878,0.605201749988751));
#11883=CARTESIAN_POINT('Ctrl Pts',(4.10000000006189,1.66887738587128,0.605315322687833));
#11884=CARTESIAN_POINT('Ctrl Pts',(4.08978435969213,1.70060618339657,-0.000163349821525811));
#11885=CARTESIAN_POINT('Ctrl Pts',(4.093189474458,1.69002990998177,0.201662875584159));
#11886=CARTESIAN_POINT('Ctrl Pts',(4.0965946873723,1.67945364446992,0.403489099757173));
#11887=CARTESIAN_POINT('Ctrl Pts',(4.1,1.66887738702936,0.605315322680078));
#11888=CARTESIAN_POINT('Ctrl Pts',(5.36191629113061,1.76821426155324,6.25990704884337E-5));
#11889=CARTESIAN_POINT('Ctrl Pts',(5.3630514496163,1.75763653340724,0.201889184585558));
#11890=CARTESIAN_POINT('Ctrl Pts',(5.36418670607087,1.74705878400967,0.403715765068683));
#11891=CARTESIAN_POINT('Ctrl Pts',(5.36532191986745,1.73648104871457,0.605542351516858));
#11892=CARTESIAN_POINT('Ctrl Pts',(6.63535348785608,1.76179300730897,3.38749616628245E-5));
#11893=CARTESIAN_POINT('Ctrl Pts',(6.63422081650235,1.75121562356675,0.20186041917081));
#11894=CARTESIAN_POINT('Ctrl Pts',(6.63308817234583,1.74063821462875,0.403686959568233));
#11895=CARTESIAN_POINT('Ctrl Pts',(6.63195543348166,1.7300608292057,0.605513504373875));
#11896=CARTESIAN_POINT('Ctrl Pts',(7.91019312949454,1.70715885937616,-0.000134060602928919));
#11897=CARTESIAN_POINT('Ctrl Pts',(7.90679525186394,1.69658223815078,0.201692207018782));
#11898=CARTESIAN_POINT('Ctrl Pts',(7.90339729485302,1.68600562209044,0.403518473580683));
#11899=CARTESIAN_POINT('Ctrl Pts',(7.89999925719352,1.67542901130525,0.605344739067286));
#11900=CARTESIAN_POINT('Origin',(3.9,1.7662962962963,0.));
#11901=CARTESIAN_POINT('',(3.9,-1.657567947596,0.605334330700044));
#11902=CARTESIAN_POINT('Ctrl Pts',(3.9,-1.657567947596,0.605334330700044));
#11903=CARTESIAN_POINT('Ctrl Pts',(3.9,-1.66295505583237,0.504667750148195));
#11904=CARTESIAN_POINT('Ctrl Pts',(3.9,-1.66834175427306,0.404000185805616));
#11905=CARTESIAN_POINT('Ctrl Pts',(3.9,-1.67913790341918,0.202222727053817));
#11906=CARTESIAN_POINT('Ctrl Pts',(3.9,-1.68454745406112,0.101110889248462));
#11907=CARTESIAN_POINT('Ctrl Pts',(3.9,-1.68995649764597,0.));
#11908=CARTESIAN_POINT('',(3.9,-1.55753217754889,0.7));
#11909=CARTESIAN_POINT('Ctrl Pts',(3.89999999700315,-1.55753217437,0.7));
#11910=CARTESIAN_POINT('Ctrl Pts',(3.89999999197785,-1.56545359401377,0.699999998841372));
#11911=CARTESIAN_POINT('Ctrl Pts',(3.90000117861029,-1.57331197233837,0.699006163267487));
#11912=CARTESIAN_POINT('Ctrl Pts',(3.90000221019459,-1.58096665047841,0.697118921400131));
#11913=CARTESIAN_POINT('Ctrl Pts',(3.90000279139136,-1.58527931230009,0.696055645348449));
#11914=CARTESIAN_POINT('Ctrl Pts',(3.90000331912093,-1.58952737074567,0.694707745526415));
#11915=CARTESIAN_POINT('Ctrl Pts',(3.90000364796674,-1.59368396010392,0.693086194530447));
#11916=CARTESIAN_POINT('Ctrl Pts',(3.90000423564848,-1.60111221870485,0.690188313817561));
#11917=CARTESIAN_POINT('Ctrl Pts',(3.90000407815102,-1.60816848972648,0.686450841450731));
#11918=CARTESIAN_POINT('Ctrl Pts',(3.9000032813392,-1.6147063365644,0.681954558458482));
#11919=CARTESIAN_POINT('Ctrl Pts',(3.90000284137901,-1.61831621321653,0.679471932695374));
#11920=CARTESIAN_POINT('Ctrl Pts',(3.90000222202081,-1.62176776859012,0.67675708350434));
#11921=CARTESIAN_POINT('Ctrl Pts',(3.9000016760669,-1.6250323621476,0.673818036286869));
#11922=CARTESIAN_POINT('Ctrl Pts',(3.90000114791654,-1.62819049732732,0.670974831382826));
#11923=CARTESIAN_POINT('Ctrl Pts',(3.90000068451114,-1.63115458712464,0.667938911589952));
#11924=CARTESIAN_POINT('Ctrl Pts',(3.90000068976928,-1.6339023205034,0.664721489040691));
#11925=CARTESIAN_POINT('Ctrl Pts',(3.90000069956116,-1.63901923218135,0.658729908073458));
#11926=CARTESIAN_POINT('Ctrl Pts',(3.9000021571807,-1.64338878348726,0.652110283780478));
#11927=CARTESIAN_POINT('Ctrl Pts',(3.90000267296827,-1.64695081636755,0.645027851744832));
#11928=CARTESIAN_POINT('Ctrl Pts',(3.90000272641596,-1.64731992654249,0.644293945625623));
#11929=CARTESIAN_POINT('Ctrl Pts',(3.90000277224081,-1.64768032438231,0.643555049900053));
#11930=CARTESIAN_POINT('Ctrl Pts',(3.90000280957334,-1.64803191324525,0.642811337026806));
#11931=CARTESIAN_POINT('Ctrl Pts',(3.90000316967295,-1.65142324611312,0.635637680016741));
#11932=CARTESIAN_POINT('Ctrl Pts',(3.90000247513984,-1.65395957542788,0.628100801230905));
#11933=CARTESIAN_POINT('Ctrl Pts',(3.90000142932204,-1.65558732484325,0.62036898832433));
#11934=CARTESIAN_POINT('Ctrl Pts',(3.90000076044003,-1.65662839749185,0.615423891207338));
#11935=CARTESIAN_POINT('Ctrl Pts',(3.9,-1.65729694754734,0.61039839235075));
#11936=CARTESIAN_POINT('Ctrl Pts',(3.9,-1.657567947596,0.605334330700044));
#11937=CARTESIAN_POINT('',(3.9,1.55753217754922,0.7));
#11938=CARTESIAN_POINT('',(3.9,0.883148148148148,0.7));
#11939=CARTESIAN_POINT('',(3.9,1.657567947596,0.605334330700044));
#11940=CARTESIAN_POINT('Ctrl Pts',(3.9,1.657567947596,0.605334330700044));
#11941=CARTESIAN_POINT('Ctrl Pts',(3.9,1.65714453107083,0.613246533660879));
#11942=CARTESIAN_POINT('Ctrl Pts',(3.90000169450566,1.65575314729854,0.621067109624563));
#11943=CARTESIAN_POINT('Ctrl Pts',(3.900002426785,1.653477907766,0.628635640467799));
#11944=CARTESIAN_POINT('Ctrl Pts',(3.90000283370343,1.65221358571927,0.632841378048222));
#11945=CARTESIAN_POINT('Ctrl Pts',(3.90000300372053,1.65067534627202,0.636969322077829));
#11946=CARTESIAN_POINT('Ctrl Pts',(3.90000288278183,1.6488710006323,0.640990000951852));
#11947=CARTESIAN_POINT('Ctrl Pts',(3.90000266510116,1.6456233127241,0.64822692378658));
#11948=CARTESIAN_POINT('Ctrl Pts',(3.90000136145047,1.64155197609259,0.655037842274187));
#11949=CARTESIAN_POINT('Ctrl Pts',(3.9000008487987,1.63672139510901,0.661259788874982));
#11950=CARTESIAN_POINT('Ctrl Pts',(3.90000075195303,1.63580884415802,0.662435184403355));
#11951=CARTESIAN_POINT('Ctrl Pts',(3.90000069125178,1.63486906637168,0.663589490553999));
#11952=CARTESIAN_POINT('Ctrl Pts',(3.90000068992127,1.63390232051248,0.664721489040685));
#11953=CARTESIAN_POINT('Ctrl Pts',(3.90000068733544,1.63202347103487,0.666921503393101));
#11954=CARTESIAN_POINT('Ctrl Pts',(3.9000009071255,1.6300427915863,0.669037305429552));
#11955=CARTESIAN_POINT('Ctrl Pts',(3.90000121037842,1.62796736695056,0.671065303566633));
#11956=CARTESIAN_POINT('Ctrl Pts',(3.90000204102081,1.62228255539437,0.676620208836154));
#11957=CARTESIAN_POINT('Ctrl Pts',(3.90000335328325,1.61595386407616,0.681456575151491));
#11958=CARTESIAN_POINT('Ctrl Pts',(3.90000380482706,1.60914557515952,0.685520902406533));
#11959=CARTESIAN_POINT('Ctrl Pts',(3.90000409284089,1.60480295930069,0.688113302965514));
#11960=CARTESIAN_POINT('Ctrl Pts',(3.90000408819389,1.6002642541482,0.690390927291682));
#11961=CARTESIAN_POINT('Ctrl Pts',(3.90000378365133,1.59556629223371,0.692330537597694));
#11962=CARTESIAN_POINT('Ctrl Pts',(3.90000330864444,1.58823869807682,0.695355823328757));
#11963=CARTESIAN_POINT('Ctrl Pts',(3.90000209726118,1.58060840086481,0.697526456028474));
#11964=CARTESIAN_POINT('Ctrl Pts',(3.90000112250675,1.5728228815436,0.698773197673241));
#11965=CARTESIAN_POINT('Ctrl Pts',(3.90000049100668,1.56777898966077,0.699580906164169));
#11966=CARTESIAN_POINT('Ctrl Pts',(3.89999999374416,1.56266934880282,0.69999999924861));
#11967=CARTESIAN_POINT('Ctrl Pts',(3.89999999700315,1.55753217437,0.7));
#11968=CARTESIAN_POINT('Ctrl Pts',(3.9,1.68995649764597,0.));
#11969=CARTESIAN_POINT('Ctrl Pts',(3.9,1.68454744095908,0.101111134163871));
#11970=CARTESIAN_POINT('Ctrl Pts',(3.9,1.67913787721413,0.202223216861756));
#11971=CARTESIAN_POINT('Ctrl Pts',(3.9,1.66834172806373,0.404000675610066));
#11972=CARTESIAN_POINT('Ctrl Pts',(3.9,1.66295504272671,0.504667995047933));
#11973=CARTESIAN_POINT('Ctrl Pts',(3.9,1.657567947596,0.605334330700044));
#11974=CARTESIAN_POINT('Ctrl Pts',(3.90000000000029,-1.68995649764598,2.25514051876985E-17));
#11975=CARTESIAN_POINT('Ctrl Pts',(3.90375240214247,-1.67935614215062,0.202290156525516));
#11976=CARTESIAN_POINT('Ctrl Pts',(3.90750491350916,-1.66875579641967,0.404580311547879));
#11977=CARTESIAN_POINT('Ctrl Pts',(3.91125753584366,-1.65815546066147,0.606870465045848));
#11978=CARTESIAN_POINT('Ctrl Pts',(2.95719731373254,-1.63434162994996,-0.000186284957671625));
#11979=CARTESIAN_POINT('Ctrl Pts',(2.96263618266967,-1.62374249289717,0.202103577800055));
#11980=CARTESIAN_POINT('Ctrl Pts',(2.96807524459186,-1.6131433886527,0.404393433349269));
#11981=CARTESIAN_POINT('Ctrl Pts',(2.97351444051957,-1.60254429060724,0.606683290324339));
#11982=CARTESIAN_POINT('Ctrl Pts',(2.0151035222252,-1.5373601393942,-0.000515615972119944));
#11983=CARTESIAN_POINT('Ctrl Pts',(2.0222299762717,-1.52676329064944,0.20177372753372));
#11984=CARTESIAN_POINT('Ctrl Pts',(2.02935668076532,-1.51616649670304,0.404063061036967));
#11985=CARTESIAN_POINT('Ctrl Pts',(2.03648357820815,-1.50556972342972,0.606352393906678));
#11986=CARTESIAN_POINT('Ctrl Pts',(1.07355614839761,-1.3885225322474,-0.00102014041634142));
#11987=CARTESIAN_POINT('Ctrl Pts',(1.08237048982668,-1.37792954541675,0.201268457136957));
#11988=CARTESIAN_POINT('Ctrl Pts',(1.09118510562603,-1.36733662501784,0.403557046289628));
#11989=CARTESIAN_POINT('Ctrl Pts',(1.09999999998551,-1.35674377243019,0.605845626932519));
#11990=CARTESIAN_POINT('Ctrl Pts',(1.10000000359112,-1.35674374984279,0.605845627045242));
#11991=CARTESIAN_POINT('Ctrl Pts',(2.02777573897866,-1.50422778688462,0.60559460123127));
#11992=CARTESIAN_POINT('Ctrl Pts',(2.96295221054883,-1.60165319397541,0.605428415101273));
#11993=CARTESIAN_POINT('Ctrl Pts',(3.9,-1.657567947596,0.605334330700044));
#11994=CARTESIAN_POINT('Ctrl Pts',(3.90594750914669,-1.55788759822396,0.7));
#11995=CARTESIAN_POINT('Ctrl Pts',(2.96654482017732,-1.50183737247472,0.7));
#11996=CARTESIAN_POINT('Ctrl Pts',(2.02939151553635,-1.40396309164617,0.7));
#11997=CARTESIAN_POINT('Ctrl Pts',(1.1,-1.25565664448621,0.7));
#11998=CARTESIAN_POINT('Ctrl Pts',(3.90422602671531,-1.58673967158186,0.7));
#11999=CARTESIAN_POINT('Ctrl Pts',(2.9639697519154,-1.53062009474021,0.699999324449154));
#12000=CARTESIAN_POINT('Ctrl Pts',(2.02587169016863,-1.43262076012027,0.700001792708215));
#12001=CARTESIAN_POINT('Ctrl Pts',(1.09546090287069,-1.28410178925883,0.700000000000001));
#12002=CARTESIAN_POINT('Ctrl Pts',(3.90124198563808,-1.6367522482393,0.676652244116846));
#12003=CARTESIAN_POINT('Ctrl Pts',(2.95951584878018,-1.58051528054544,0.676683243227538));
#12004=CARTESIAN_POINT('Ctrl Pts',(2.01975879699698,-1.48229505764113,0.676737195552829));
#12005=CARTESIAN_POINT('Ctrl Pts',(1.08759175402576,-1.33341535796084,0.676819902351873));
#12006=CARTESIAN_POINT('Ctrl Pts',(3.90006887217438,-1.65641364884095,0.626981005337021));
#12007=CARTESIAN_POINT('Ctrl Pts',(2.95775794493813,-1.6001648299169,0.627061170854983));
#12008=CARTESIAN_POINT('Ctrl Pts',(2.01735267249256,-1.50192280897576,0.627202240820629));
#12009=CARTESIAN_POINT('Ctrl Pts',(1.08446813262788,-1.35299014570964,0.627416665943555));
#12010=CARTESIAN_POINT('Ctrl Pts',(3.9,-1.657567947596,0.605334330700044));
#12011=CARTESIAN_POINT('Ctrl Pts',(2.95765589353472,-1.60133715645388,0.605428946878649));
#12012=CARTESIAN_POINT('Ctrl Pts',(2.01720431860088,-1.50312513840151,0.605596482146283));
#12013=CARTESIAN_POINT('Ctrl Pts',(1.0842689834292,-1.35423815332579,0.605849891671036));
#12014=CARTESIAN_POINT('Ctrl Pts',(3.89999999700313,-1.55753217437,0.7));
#12015=CARTESIAN_POINT('Ctrl Pts',(2.96258932077475,-1.50142404037792,0.7));
#12016=CARTESIAN_POINT('Ctrl Pts',(2.02743012901897,-1.40365010593343,0.7));
#12017=CARTESIAN_POINT('Ctrl Pts',(1.1,-1.25565664448621,0.7));
#12018=CARTESIAN_POINT('Origin',(6.08012166120517,1.06778195214465E-16,
0.7));
#12019=CARTESIAN_POINT('Ctrl Pts',(1.1,1.25565664448621,0.7));
#12020=CARTESIAN_POINT('Ctrl Pts',(2.02743012901899,1.40365010593344,0.7));
#12021=CARTESIAN_POINT('Ctrl Pts',(2.96258932077472,1.50142404037792,0.7));
#12022=CARTESIAN_POINT('Ctrl Pts',(3.89999999700315,1.55753217437,0.7));
#12023=CARTESIAN_POINT('Ctrl Pts',(1.1,1.25565664448621,0.7));
#12024=CARTESIAN_POINT('Ctrl Pts',(2.02939151553637,1.40396309164617,0.7));
#12025=CARTESIAN_POINT('Ctrl Pts',(2.96654482017727,1.50183737247472,0.7));
#12026=CARTESIAN_POINT('Ctrl Pts',(3.90594750914669,1.55788759822396,0.7));
#12027=CARTESIAN_POINT('Ctrl Pts',(1.09546090287069,1.28410178925883,0.700000000000001));
#12028=CARTESIAN_POINT('Ctrl Pts',(2.02587169016866,1.43262076012027,0.700001792708215));
#12029=CARTESIAN_POINT('Ctrl Pts',(2.96396975191535,1.53062009474021,0.699999324449154));
#12030=CARTESIAN_POINT('Ctrl Pts',(3.90422602671531,1.58673967158186,0.7));
#12031=CARTESIAN_POINT('Ctrl Pts',(1.08759175402576,1.33341535796084,0.676819902351873));
#12032=CARTESIAN_POINT('Ctrl Pts',(2.019758796997,1.48229505764113,0.676737195552829));
#12033=CARTESIAN_POINT('Ctrl Pts',(2.95951584878014,1.58051528054544,0.676683243227538));
#12034=CARTESIAN_POINT('Ctrl Pts',(3.90124198563808,1.6367522482393,0.676652244116846));
#12035=CARTESIAN_POINT('Ctrl Pts',(1.08446813262788,1.35299014570964,0.627416665943555));
#12036=CARTESIAN_POINT('Ctrl Pts',(2.01735267249258,1.50192280897576,0.627202240820629));
#12037=CARTESIAN_POINT('Ctrl Pts',(2.95775794493809,1.6001648299169,0.627061170854983));
#12038=CARTESIAN_POINT('Ctrl Pts',(3.90006887217438,1.65641364884095,0.626981005337021));
#12039=CARTESIAN_POINT('Ctrl Pts',(1.0842689834292,1.35423815332579,0.605849891671036));
#12040=CARTESIAN_POINT('Ctrl Pts',(2.0172043186009,1.50312513840152,0.605596482146283));
#12041=CARTESIAN_POINT('Ctrl Pts',(2.95765589353468,1.60133715645387,0.605428946878649));
#12042=CARTESIAN_POINT('Ctrl Pts',(3.9,1.657567947596,0.605334330700044));
#12043=CARTESIAN_POINT('Ctrl Pts',(3.9,1.657567947596,0.605334330700044));
#12044=CARTESIAN_POINT('Ctrl Pts',(2.96295221054879,1.60165319397541,0.605428415101273));
#12045=CARTESIAN_POINT('Ctrl Pts',(2.02777573897867,1.50422778688462,0.60559460123127));
#12046=CARTESIAN_POINT('Ctrl Pts',(1.10000000359111,1.35674374984279,0.605845627045242));
#12047=CARTESIAN_POINT('Ctrl Pts',(1.07355614839761,1.3885225322474,-0.00102014041634139));
#12048=CARTESIAN_POINT('Ctrl Pts',(1.08237048982668,1.37792954541676,0.201268457136957));
#12049=CARTESIAN_POINT('Ctrl Pts',(1.09118510562602,1.36733662501784,0.403557046289628));
#12050=CARTESIAN_POINT('Ctrl Pts',(1.09999999998551,1.35674377243019,0.605845626932519));
#12051=CARTESIAN_POINT('Ctrl Pts',(2.0151035222252,1.5373601393942,-0.000515615972119942));
#12052=CARTESIAN_POINT('Ctrl Pts',(2.0222299762717,1.52676329064944,0.201773727533721));
#12053=CARTESIAN_POINT('Ctrl Pts',(2.02935668076532,1.51616649670304,0.404063061036968));
#12054=CARTESIAN_POINT('Ctrl Pts',(2.03648357820815,1.50556972342972,0.606352393906678));
#12055=CARTESIAN_POINT('Ctrl Pts',(2.95719731373254,1.63434162994996,-0.000186284957671606));
#12056=CARTESIAN_POINT('Ctrl Pts',(2.96263618266967,1.62374249289717,0.202103577800055));
#12057=CARTESIAN_POINT('Ctrl Pts',(2.96807524459186,1.6131433886527,0.404393433349269));
#12058=CARTESIAN_POINT('Ctrl Pts',(2.97351444051957,1.60254429060724,0.60668329032434));
#12059=CARTESIAN_POINT('Ctrl Pts',(3.90000000000029,1.68995649764598,4.33680868994202E-17));
#12060=CARTESIAN_POINT('Ctrl Pts',(3.90375240214247,1.67935614215062,0.202290156525516));
#12061=CARTESIAN_POINT('Ctrl Pts',(3.90750491350917,1.66875579641967,0.404580311547879));
#12062=CARTESIAN_POINT('Ctrl Pts',(3.91125753584366,1.65815546066147,0.606870465045848));
#12063=CARTESIAN_POINT('Origin',(0.9,1.44962962962963,0.));
#12064=CARTESIAN_POINT('',(0.900000000000025,-1.32415632515176,0.605901073595307));
#12065=CARTESIAN_POINT('Ctrl Pts',(0.900000000000025,-1.32415632515176,
0.605901073595307));
#12066=CARTESIAN_POINT('Ctrl Pts',(0.900000000000025,-1.33021622058432,
0.504787384877132));
#12067=CARTESIAN_POINT('Ctrl Pts',(0.900000000000001,-1.33627289299046,
0.403672458220672));
#12068=CARTESIAN_POINT('Ctrl Pts',(0.900000000000001,-1.3483639425303,0.201706128802639));
#12069=CARTESIAN_POINT('Ctrl Pts',(0.9,-1.3543984610184,0.100852646477479));
#12070=CARTESIAN_POINT('Ctrl Pts',(0.9,-1.3604297237941,0.));
#12071=CARTESIAN_POINT('',(0.9,-1.22294421121193,0.7));
#12072=CARTESIAN_POINT('Ctrl Pts',(0.899999998934589,-1.2229442093848,0.7));
#12073=CARTESIAN_POINT('Ctrl Pts',(0.89999998269596,-1.2309559991361,0.699999991698178));
#12074=CARTESIAN_POINT('Ctrl Pts',(0.900003161357076,-1.2389110096839,0.699008412490225));
#12075=CARTESIAN_POINT('Ctrl Pts',(0.900005837532895,-1.24666554379878,
0.697120920272419));
#12076=CARTESIAN_POINT('Ctrl Pts',(0.900007138246235,-1.25043451364619,
0.69620353424371));
#12077=CARTESIAN_POINT('Ctrl Pts',(0.900008321383585,-1.25415610217771,
0.695073675615989));
#12078=CARTESIAN_POINT('Ctrl Pts',(0.900009136546862,-1.25781268161099,
0.69373809091454));
#12079=CARTESIAN_POINT('Ctrl Pts',(0.90001081442992,-1.26533916477404,0.690989003700189));
#12080=CARTESIAN_POINT('Ctrl Pts',(0.900010659344479,-1.27251458345821,
0.687399440976464));
#12081=CARTESIAN_POINT('Ctrl Pts',(0.900008585023094,-1.27919110928202,
0.68304500924512));
#12082=CARTESIAN_POINT('Ctrl Pts',(0.900007251085311,-1.28348459539356,
0.680244796581297));
#12083=CARTESIAN_POINT('Ctrl Pts',(0.900005156998288,-1.28757155292352,
0.67712723751572));
#12084=CARTESIAN_POINT('Ctrl Pts',(0.900003422242992,-1.29140570811059,
0.673703384872626));
#12085=CARTESIAN_POINT('Ctrl Pts',(0.90000203719427,-1.29446694202502,0.670969741262059));
#12086=CARTESIAN_POINT('Ctrl Pts',(0.90000088611098,-1.29734878548314,0.668056850549005));
#12087=CARTESIAN_POINT('Ctrl Pts',(0.900000936626746,-1.30003070819003,
0.664973821719563));
#12088=CARTESIAN_POINT('Ctrl Pts',(0.90000103432908,-1.30521780373233,0.659010948495488));
#12089=CARTESIAN_POINT('Ctrl Pts',(0.900005119671874,-1.30966005175478,
0.652412896960716));
#12090=CARTESIAN_POINT('Ctrl Pts',(0.900006662646281,-1.31329014967729,
0.64534035177384));
#12091=CARTESIAN_POINT('Ctrl Pts',(0.900006837929091,-1.31370253096037,
0.644536906434065));
#12092=CARTESIAN_POINT('Ctrl Pts',(0.900006988901759,-1.3141043809937,0.64372731654354));
#12093=CARTESIAN_POINT('Ctrl Pts',(0.900007112770807,-1.31449556093743,
0.642911804846506));
#12094=CARTESIAN_POINT('Ctrl Pts',(0.900008198175579,-1.31792328224658,
0.635765868899185));
#12095=CARTESIAN_POINT('Ctrl Pts',(0.900006415208278,-1.32049402672979,
0.628253543462219));
#12096=CARTESIAN_POINT('Ctrl Pts',(0.900003664797616,-1.32215034643222,
0.620540220943237));
#12097=CARTESIAN_POINT('Ctrl Pts',(0.900001948338234,-1.32318401225236,
0.615726538031782));
#12098=CARTESIAN_POINT('Ctrl Pts',(0.900000000000001,-1.32386068836271,
0.610833984830158));
#12099=CARTESIAN_POINT('Ctrl Pts',(0.900000000000001,-1.32415632515176,
0.605901073595307));
#12100=CARTESIAN_POINT('',(0.9,1.22294421121193,0.7));
#12101=CARTESIAN_POINT('',(0.9,0.724814814814815,0.7));
#12102=CARTESIAN_POINT('',(0.900000000000027,1.32415632515176,0.605901073595307));
#12103=CARTESIAN_POINT('Ctrl Pts',(0.900000000000001,1.32415632515176,0.605901073595307));
#12104=CARTESIAN_POINT('Ctrl Pts',(0.900000000000001,1.32368299187747,0.613798977756921));
#12105=CARTESIAN_POINT('Ctrl Pts',(0.900004523569871,1.32223544152535,0.621596324701597));
#12106=CARTESIAN_POINT('Ctrl Pts',(0.900006356724635,1.31990036466821,0.629134362570908));
#12107=CARTESIAN_POINT('Ctrl Pts',(0.900007328861843,1.3186620540024,0.633131846706937));
#12108=CARTESIAN_POINT('Ctrl Pts',(0.900007702029268,1.31717322147439,0.637056437951431));
#12109=CARTESIAN_POINT('Ctrl Pts',(0.900007358328755,1.31544117393516,0.640882963165587));
#12110=CARTESIAN_POINT('Ctrl Pts',(0.900006707239278,1.31216006761937,0.648131745755711));
#12111=CARTESIAN_POINT('Ctrl Pts',(0.900003091243194,1.3080468004769,0.654946293188228));
#12112=CARTESIAN_POINT('Ctrl Pts',(0.900001489347898,1.30317324258861,0.661167512355852));
#12113=CARTESIAN_POINT('Ctrl Pts',(0.900001155878064,1.30215870403359,0.662462596327245));
#12114=CARTESIAN_POINT('Ctrl Pts',(0.90000093695446,1.30111105636563,0.663731893727214));
#12115=CARTESIAN_POINT('Ctrl Pts',(0.90000091848414,1.30003070515708,0.664973821721807));
#12116=CARTESIAN_POINT('Ctrl Pts',(0.90000089007412,1.29836896897911,0.666884086330845));
#12117=CARTESIAN_POINT('Ctrl Pts',(0.900001333486324,1.29662987445651,0.668729618924651));
#12118=CARTESIAN_POINT('Ctrl Pts',(0.900001997973453,1.2948182721625,0.670508241825176));
#12119=CARTESIAN_POINT('Ctrl Pts',(0.900004083621534,1.28913213515815,0.676090865298813));
#12120=CARTESIAN_POINT('Ctrl Pts',(0.900007925915178,1.28279871831387,0.680954424681199));
#12121=CARTESIAN_POINT('Ctrl Pts',(0.900009431597099,1.27598654051802,0.685053039288488));
#12122=CARTESIAN_POINT('Ctrl Pts',(0.900010426918848,1.2714833923965,0.687762403198649));
#12123=CARTESIAN_POINT('Ctrl Pts',(0.900010579450444,1.26676996242859,0.690136867340003));
#12124=CARTESIAN_POINT('Ctrl Pts',(0.900009885932263,1.26188774903006,0.692153145632694));
#12125=CARTESIAN_POINT('Ctrl Pts',(0.900008832351734,1.25447077696631,0.695216239878874));
#12126=CARTESIAN_POINT('Ctrl Pts',(0.900005746465811,1.24674633448708,0.697421320974322));
#12127=CARTESIAN_POINT('Ctrl Pts',(0.900003140090462,1.23886595492982,0.6987028844583));
#12128=CARTESIAN_POINT('Ctrl Pts',(0.900001403206082,1.23361448254879,0.699556916322089));
#12129=CARTESIAN_POINT('Ctrl Pts',(0.899999988093253,1.22829309040712,0.699999994457486));
#12130=CARTESIAN_POINT('Ctrl Pts',(0.899999998934588,1.2229442093848,0.7));
#12131=CARTESIAN_POINT('Ctrl Pts',(0.9,1.3604297237941,0.));
#12132=CARTESIAN_POINT('Ctrl Pts',(0.9,1.35439838926384,0.100853846331769));
#12133=CARTESIAN_POINT('Ctrl Pts',(0.9,1.34836379894337,0.201708528537181));
#12134=CARTESIAN_POINT('Ctrl Pts',(0.9,1.33627274925098,0.403674857922336));
#12135=CARTESIAN_POINT('Ctrl Pts',(0.900000000000027,1.33021614867672,0.504788584706939));
#12136=CARTESIAN_POINT('Ctrl Pts',(0.900000000000027,1.32415632515176,0.605901073595307));
#12137=CARTESIAN_POINT('Ctrl Pts',(0.900000000000001,-1.3604297237941,-1.73472347597681E-18));
#12138=CARTESIAN_POINT('Ctrl Pts',(0.909119345746934,-1.34984469470005,
0.202150401646216));
#12139=CARTESIAN_POINT('Ctrl Pts',(0.918238975454288,-1.33925973741039,
0.404300794324169));
#12140=CARTESIAN_POINT('Ctrl Pts',(0.92735889343571,-1.32867485341111,0.606451177918334));
#12141=CARTESIAN_POINT('Ctrl Pts',(0.693791632045388,-1.32642527651154,
-0.000115194085079675));
#12142=CARTESIAN_POINT('Ctrl Pts',(0.703280422539661,-1.31584113310577,
0.202035038813999));
#12143=CARTESIAN_POINT('Ctrl Pts',(0.712769508818954,-1.30525706820637,
0.404185262036053));
#12144=CARTESIAN_POINT('Ctrl Pts',(0.722258895242942,-1.29467308328318,
0.606335475483814));
#12145=CARTESIAN_POINT('Ctrl Pts',(0.487608314405001,-1.28990207050556,
-0.000238777108575344));
#12146=CARTESIAN_POINT('Ctrl Pts',(0.497466558273561,-1.27931888757273,
0.201911276725417));
#12147=CARTESIAN_POINT('Ctrl Pts',(0.507325109482935,-1.26873579028159,
0.404061320158324));
#12148=CARTESIAN_POINT('Ctrl Pts',(0.517183972542757,-1.25815278023897,
0.606211353085106));
#12149=CARTESIAN_POINT('Ctrl Pts',(0.281447431601629,-1.2507496025167,-0.000370926150909055));
#12150=CARTESIAN_POINT('Ctrl Pts',(0.291675125201343,-1.24016745708839,
0.201778938960696));
#12151=CARTESIAN_POINT('Ctrl Pts',(0.301903137322998,-1.2295854048496,0.403928792940867));
#12152=CARTESIAN_POINT('Ctrl Pts',(0.312131472716966,-1.21900344770756,
0.606078635650713));
#12153=CARTESIAN_POINT('',(0.313137632044026,-1.21919552599285,0.606079286803921));
#12154=CARTESIAN_POINT('Ctrl Pts',(0.28146619846596,-1.25073018526678,-6.36968776335234E-17));
#12155=CARTESIAN_POINT('Ctrl Pts',(0.292023490345879,-1.2402182973453,0.20202640462578));
#12156=CARTESIAN_POINT('Ctrl Pts',(0.302580635585432,-1.22970674279184,
0.404052833452346));
#12157=CARTESIAN_POINT('Ctrl Pts',(0.313137632044028,-1.21919552599286,
0.606079286803922));
#12158=CARTESIAN_POINT('Ctrl Pts',(0.313137632044026,-1.21919552599285,
0.606079286803921));
#12159=CARTESIAN_POINT('Ctrl Pts',(0.508347756773358,-1.25646926692181,
0.606016122348466));
#12160=CARTESIAN_POINT('Ctrl Pts',(0.703992099548353,-1.29143758865737,
0.605956720831638));
#12161=CARTESIAN_POINT('Ctrl Pts',(0.900000000000031,-1.32415632515176,
0.605901073595307));
#12162=CARTESIAN_POINT('Ctrl Pts',(0.916434425702686,-1.22569269236154,
0.7));
#12163=CARTESIAN_POINT('Ctrl Pts',(0.72117838049967,-1.193102781986,0.7));
#12164=CARTESIAN_POINT('Ctrl Pts',(0.526295996270969,-1.15827411715321,
0.7));
#12165=CARTESIAN_POINT('Ctrl Pts',(0.3318563713692,-1.12115139781564,0.7));
#12166=CARTESIAN_POINT('Ctrl Pts',(0.911693828447622,-1.25409504944868,
0.700000000000001));
#12167=CARTESIAN_POINT('Ctrl Pts',(0.716221724293519,-1.22145811194286,
0.699999606692487));
#12168=CARTESIAN_POINT('Ctrl Pts',(0.52112301919326,-1.18657973614434,0.700000445015345));
#12169=CARTESIAN_POINT('Ctrl Pts',(0.32646265058614,-1.14940237362229,0.699999999999999));
#12170=CARTESIAN_POINT('Ctrl Pts',(0.903473253113197,-1.30334701150065,
0.676847307332805));
#12171=CARTESIAN_POINT('Ctrl Pts',(0.707628846166824,-1.27063023858114,
0.676865462359186));
#12172=CARTESIAN_POINT('Ctrl Pts',(0.512149925983835,-1.23566412474798,
0.676884474751893));
#12173=CARTESIAN_POINT('Ctrl Pts',(0.317109102097966,-1.19839394783867,
0.676905055067496));
#12174=CARTESIAN_POINT('Ctrl Pts',(0.900209809599689,-1.32289929215588,
0.627459885485154));
#12175=CARTESIAN_POINT('Ctrl Pts',(0.704212910592823,-1.29017057588713,
0.627506965865002));
#12176=CARTESIAN_POINT('Ctrl Pts',(0.50858160780484,-1.25519230329596,0.627556915196293));
#12177=CARTESIAN_POINT('Ctrl Pts',(0.31338355686088,-1.21790743260971,0.627610331402299));
#12178=CARTESIAN_POINT('Ctrl Pts',(0.900000000000031,-1.32415632515176,
0.605901073595307));
#12179=CARTESIAN_POINT('Ctrl Pts',(0.703992099548353,-1.29143758865737,
0.605956720831638));
#12180=CARTESIAN_POINT('Ctrl Pts',(0.508347756773358,-1.25646926692181,
0.606016122348466));
#12181=CARTESIAN_POINT('Ctrl Pts',(0.313137632044026,-1.21919552599285,
0.606079286803921));
#12182=CARTESIAN_POINT('',(0.3318563713692,-1.12115139781563,0.7));
#12183=CARTESIAN_POINT('Origin',(0.331856371369202,-1.12115139781563,0.6));
#12184=CARTESIAN_POINT('Ctrl Pts',(0.899999998934586,-1.2229442093848,0.7));
#12185=CARTESIAN_POINT('Ctrl Pts',(0.71024282334811,-1.19114655107378,0.7));
#12186=CARTESIAN_POINT('Ctrl Pts',(0.520840466228891,-1.15723253876768,
0.7));
#12187=CARTESIAN_POINT('Ctrl Pts',(0.3318563713692,-1.12115139781564,0.7));
#12188=CARTESIAN_POINT('Origin',(6.08012166120517,1.06778195214465E-16,
0.7));
#12189=CARTESIAN_POINT('',(0.331856371369203,1.12115139781563,0.7));
#12190=CARTESIAN_POINT('',(0.3318563713692,-0.7,0.7));
#12191=CARTESIAN_POINT('Ctrl Pts',(0.331856371369202,1.12115139781564,0.7));
#12192=CARTESIAN_POINT('Ctrl Pts',(0.520840466228894,1.15723253876768,0.7));
#12193=CARTESIAN_POINT('Ctrl Pts',(0.710242823348114,1.19114655107378,0.7));
#12194=CARTESIAN_POINT('Ctrl Pts',(0.899999998934589,1.2229442093848,0.7));
#12195=CARTESIAN_POINT('Ctrl Pts',(0.281447431601628,1.2507496025167,-0.000370926150909064));
#12196=CARTESIAN_POINT('Ctrl Pts',(0.291675125201342,1.24016745708839,0.201778938960695));
#12197=CARTESIAN_POINT('Ctrl Pts',(0.301903137322998,1.2295854048496,0.403928792940867));
#12198=CARTESIAN_POINT('Ctrl Pts',(0.312131472716965,1.21900344770756,0.606078635650713));
#12199=CARTESIAN_POINT('Ctrl Pts',(0.487608314405001,1.28990207050556,-0.000238777108575355));
#12200=CARTESIAN_POINT('Ctrl Pts',(0.497466558273561,1.27931888757273,0.201911276725417));
#12201=CARTESIAN_POINT('Ctrl Pts',(0.507325109482935,1.26873579028159,0.404061320158324));
#12202=CARTESIAN_POINT('Ctrl Pts',(0.517183972542757,1.25815278023897,0.606211353085106));
#12203=CARTESIAN_POINT('Ctrl Pts',(0.693791632045388,1.32642527651154,-0.000115194085079627));
#12204=CARTESIAN_POINT('Ctrl Pts',(0.703280422539661,1.31584113310577,0.202035038813999));
#12205=CARTESIAN_POINT('Ctrl Pts',(0.712769508818955,1.30525706820637,0.404185262036054));
#12206=CARTESIAN_POINT('Ctrl Pts',(0.722258895242942,1.29467308328318,0.606335475483814));
#12207=CARTESIAN_POINT('Ctrl Pts',(0.900000000000002,1.3604297237941,4.33680868994202E-17));
#12208=CARTESIAN_POINT('Ctrl Pts',(0.909119345746935,1.34984469470005,0.202150401646216));
#12209=CARTESIAN_POINT('Ctrl Pts',(0.918238975454289,1.33925973741039,0.40430079432417));
#12210=CARTESIAN_POINT('Ctrl Pts',(0.927358893435711,1.32867485341111,0.606451177918334));
#12211=CARTESIAN_POINT('',(0.313137632044028,1.21919552599286,0.606079286803921));
#12212=CARTESIAN_POINT('Ctrl Pts',(0.900000000000026,1.32415632515176,0.605901073595307));
#12213=CARTESIAN_POINT('Ctrl Pts',(0.703992099548352,1.29143758865737,0.605956720831638));
#12214=CARTESIAN_POINT('Ctrl Pts',(0.508347756773358,1.25646926692181,0.606016122348466));
#12215=CARTESIAN_POINT('Ctrl Pts',(0.313137632044028,1.21919552599286,0.606079286803921));
#12216=CARTESIAN_POINT('Ctrl Pts',(0.313137632044028,1.21919552599286,0.606079286803922));
#12217=CARTESIAN_POINT('Ctrl Pts',(0.302580635585432,1.22970674279184,0.404052833452346));
#12218=CARTESIAN_POINT('Ctrl Pts',(0.29202349034588,1.2402182973453,0.20202640462578));
#12219=CARTESIAN_POINT('Ctrl Pts',(0.28146619846596,1.25073018526678,-6.5594231435373E-18));
#12220=CARTESIAN_POINT('Ctrl Pts',(0.331856371369202,1.12115139781564,0.7));
#12221=CARTESIAN_POINT('Ctrl Pts',(0.526295996270969,1.15827411715321,0.7));
#12222=CARTESIAN_POINT('Ctrl Pts',(0.72117838049967,1.193102781986,0.7));
#12223=CARTESIAN_POINT('Ctrl Pts',(0.916434425702682,1.22569269236154,0.7));
#12224=CARTESIAN_POINT('Ctrl Pts',(0.326462650586141,1.14940237362229,0.699999999999999));
#12225=CARTESIAN_POINT('Ctrl Pts',(0.52112301919326,1.18657973614434,0.700000445015345));
#12226=CARTESIAN_POINT('Ctrl Pts',(0.716221724293519,1.22145811194286,0.699999606692487));
#12227=CARTESIAN_POINT('Ctrl Pts',(0.911693828447618,1.25409504944868,0.700000000000001));
#12228=CARTESIAN_POINT('Ctrl Pts',(0.317109102097967,1.19839394783867,0.676905055067496));
#12229=CARTESIAN_POINT('Ctrl Pts',(0.512149925983836,1.23566412474798,0.676884474751893));
#12230=CARTESIAN_POINT('Ctrl Pts',(0.707628846166824,1.27063023858114,0.676865462359185));
#12231=CARTESIAN_POINT('Ctrl Pts',(0.903473253113193,1.30334701150065,0.676847307332805));
#12232=CARTESIAN_POINT('Ctrl Pts',(0.313383556860882,1.21790743260971,0.627610331402299));
#12233=CARTESIAN_POINT('Ctrl Pts',(0.508581607804839,1.25519230329596,0.627556915196293));
#12234=CARTESIAN_POINT('Ctrl Pts',(0.704212910592822,1.29017057588713,0.627506965865002));
#12235=CARTESIAN_POINT('Ctrl Pts',(0.900209809599685,1.32289929215587,0.627459885485154));
#12236=CARTESIAN_POINT('Ctrl Pts',(0.313137632044028,1.21919552599286,0.606079286803921));
#12237=CARTESIAN_POINT('Ctrl Pts',(0.508347756773358,1.25646926692181,0.606016122348466));
#12238=CARTESIAN_POINT('Ctrl Pts',(0.703992099548352,1.29143758865737,0.605956720831638));
#12239=CARTESIAN_POINT('Ctrl Pts',(0.900000000000026,1.32415632515176,0.605901073595307));
#12240=CARTESIAN_POINT('Origin',(0.3318563713692,1.12115139781563,0.6));
#12241=CARTESIAN_POINT('Origin',(0.3318563713692,1.12115139781563,0.6));
#12242=CARTESIAN_POINT('Origin',(0.3318563713692,1.12115139781563,0.6));
#12243=CARTESIAN_POINT('Origin',(0.331856371369201,1.12115139781563,0.6));
#12244=CARTESIAN_POINT('Origin',(11.6681436286308,1.2964346619681,0.6));
#12245=CARTESIAN_POINT('Origin',(11.6681436286308,1.2964346619681,0.6));
#12246=CARTESIAN_POINT('',(11.7680065821063,1.2964346619681,0.605233595624295));
#12247=CARTESIAN_POINT('Origin',(11.6681436286308,1.2964346619681,0.6));
#12248=CARTESIAN_POINT('Origin',(11.6681436286308,1.2964346619681,0.6));
#12249=CARTESIAN_POINT('Origin',(0.3318563713692,-1.12115139781563,0.6));
#12250=CARTESIAN_POINT('Origin',(0.3318563713692,-1.12115139781563,0.6));
#12251=CARTESIAN_POINT('Origin',(0.3318563713692,-1.12115139781563,0.6));
#12252=CARTESIAN_POINT('Origin',(0.3318563713692,-0.7,0.6));
#12253=CARTESIAN_POINT('Ctrl Pts',(0.281398851089427,-1.25079724300364,
-0.00128877254616805));
#12254=CARTESIAN_POINT('Ctrl Pts',(0.291978592719145,-1.24026300108396,
0.201167222825305));
#12255=CARTESIAN_POINT('Ctrl Pts',(0.302558187088771,-1.2297290939422,0.403623242499903));
#12256=CARTESIAN_POINT('Ctrl Pts',(0.313137632044028,-1.21919552599286,
0.606079286803922));
#12257=CARTESIAN_POINT('Ctrl Pts',(0.258825925396095,-1.24645021448495,
-0.000331836826913007));
#12258=CARTESIAN_POINT('Ctrl Pts',(0.269412087408768,-1.23590982471973,
0.202123507634926));
#12259=CARTESIAN_POINT('Ctrl Pts',(0.279998097240749,-1.22537010804418,
0.404578894752494));
#12260=CARTESIAN_POINT('Ctrl Pts',(0.290584031570127,-1.21483034200885,
0.60703428203898));
#12261=CARTESIAN_POINT('Ctrl Pts',(0.216858515231733,-1.22156435206688,
0.000573427186746937));
#12262=CARTESIAN_POINT('Ctrl Pts',(0.22746089442761,-1.21102065820065,0.20302778119957));
#12263=CARTESIAN_POINT('Ctrl Pts',(0.238063405890532,-1.20047706879609,
0.405482132943502));
#12264=CARTESIAN_POINT('Ctrl Pts',(0.248665715176951,-1.18993398276804,
0.607936521147589));
#12265=CARTESIAN_POINT('Ctrl Pts',(0.20022524016831,-1.1757120364715,-0.000939345874739115));
#12266=CARTESIAN_POINT('Ctrl Pts',(0.210835545796271,-1.16517845930889,
0.201515175954065));
#12267=CARTESIAN_POINT('Ctrl Pts',(0.221445511453644,-1.15464532122135,
0.403969738345816));
#12268=CARTESIAN_POINT('Ctrl Pts',(0.232055819885544,-1.1441124535127,0.606424296559432));
#12269=CARTESIAN_POINT('Ctrl Pts',(0.200162791320387,-1.15273540576203,
-0.00213094087794781));
#12270=CARTESIAN_POINT('Ctrl Pts',(0.210772999146098,-1.14220702337553,
0.200323884929633));
#12271=CARTESIAN_POINT('Ctrl Pts',(0.221383207999129,-1.13167901896849,
0.402778730339676));
#12272=CARTESIAN_POINT('Ctrl Pts',(0.231993417893744,-1.12115139781563,
0.605233595624295));
#12273=CARTESIAN_POINT('Origin',(11.6681436286308,-1.2964346619681,0.6));
#12274=CARTESIAN_POINT('',(11.7680065821063,-1.2964346619681,0.605233595624295));
#12275=CARTESIAN_POINT('Origin',(11.6681436286308,-1.2964346619681,0.6));
#12276=CARTESIAN_POINT('Origin',(11.6681436286308,-1.2964346619681,0.6));
#12277=CARTESIAN_POINT('Origin',(11.6681436286308,0.8,0.6));
#12278=CARTESIAN_POINT('',(11.7680065821063,0.8,0.605233595624295));
#12279=CARTESIAN_POINT('Ctrl Pts',(11.7998406965532,-1.32812796269332,-0.00219749346969486));
#12280=CARTESIAN_POINT('Ctrl Pts',(11.7892293257052,-1.31756329650235,0.200279524124498));
#12281=CARTESIAN_POINT('Ctrl Pts',(11.778617954226,-1.30699886176745,0.402756553762325));
#12282=CARTESIAN_POINT('Ctrl Pts',(11.7680065821063,-1.2964346619681,0.605233595624295));
#12283=CARTESIAN_POINT('Ctrl Pts',(11.7997644051931,-1.35610429277321,-0.000741767599518841));
#12284=CARTESIAN_POINT('Ctrl Pts',(11.7891529352516,-1.34553639595159,0.201735054786578));
#12285=CARTESIAN_POINT('Ctrl Pts',(11.7785417923834,-1.33496887357233,0.404211913913734));
#12286=CARTESIAN_POINT('Ctrl Pts',(11.7679303202531,-1.32440140973518,0.606688758469115));
#12287=CARTESIAN_POINT('Ctrl Pts',(11.777798894316,-1.40464673224301,0.000639873095493681));
#12288=CARTESIAN_POINT('Ctrl Pts',(11.7671928076068,-1.39407357725403,0.203116666245104));
#12289=CARTESIAN_POINT('Ctrl Pts',(11.7565866683578,-1.38350056680667,0.405593463707878));
#12290=CARTESIAN_POINT('Ctrl Pts',(11.7459806329718,-1.37292778989405,0.608070278434593));
#12291=CARTESIAN_POINT('Ctrl Pts',(11.7305637688674,-1.42539741767755,-0.000752904078362463));
#12292=CARTESIAN_POINT('Ctrl Pts',(11.7199663219939,-1.4148278080644,0.201724510929383));
#12293=CARTESIAN_POINT('Ctrl Pts',(11.7093688723049,-1.40425849106451,0.404201940657439));
#12294=CARTESIAN_POINT('Ctrl Pts',(11.6987715660822,-1.39368929079062,0.606679383299034));
#12295=CARTESIAN_POINT('Ctrl Pts',(11.7096810564041,-1.4274931182575,-0.0017379730583696));
#12296=CARTESIAN_POINT('Ctrl Pts',(11.6990862989954,-1.41692678914967,0.200739752511227));
#12297=CARTESIAN_POINT('Ctrl Pts',(11.6884916259906,-1.40636067879325,0.403217493356832));
#12298=CARTESIAN_POINT('Ctrl Pts',(11.6778970386953,-1.39579479040469,0.605695249702977));
#12299=CARTESIAN_POINT('Ctrl Pts',(11.7997255308004,-1.32801330383774,1.58293517182884E-17));
#12300=CARTESIAN_POINT('Ctrl Pts',(11.7891525485321,-1.31748685893698,0.201744519857947));
#12301=CARTESIAN_POINT('Ctrl Pts',(11.7785795656372,-1.30696064383315,0.403489051673192));
#12302=CARTESIAN_POINT('Ctrl Pts',(11.7680065821063,-1.2964346619681,0.605233595624295));
#12303=CARTESIAN_POINT('Ctrl Pts',(11.7096782931395,1.42749036240749,-0.00168516396645821));
#12304=CARTESIAN_POINT('Ctrl Pts',(11.6990844568337,1.41692495195436,0.200774958575157));
#12305=CARTESIAN_POINT('Ctrl Pts',(11.6884907049172,1.40635976021489,0.403235096390144));
#12306=CARTESIAN_POINT('Ctrl Pts',(11.6778970386953,1.39579479040469,0.605695249702978));
#12307=CARTESIAN_POINT('Ctrl Pts',(11.7375219088137,1.42469609383707,-0.000371738767665111));
#12308=CARTESIAN_POINT('Ctrl Pts',(11.7269244310859,1.41412622652679,0.202087962343291));
#12309=CARTESIAN_POINT('Ctrl Pts',(11.7163270893473,1.40355692684423,0.404547700208143));
#12310=CARTESIAN_POINT('Ctrl Pts',(11.7057297418778,1.39298745758592,0.607007427831054));
#12311=CARTESIAN_POINT('Ctrl Pts',(11.7837126264455,1.39812338730171,0.000662527065309348));
#12312=CARTESIAN_POINT('Ctrl Pts',(11.7731059659782,1.38755170250994,0.203121672627585));
#12313=CARTESIAN_POINT('Ctrl Pts',(11.762499302106,1.37698011891703,0.405580822779681));
#12314=CARTESIAN_POINT('Ctrl Pts',(11.7518926781287,1.36640881816393,0.608039989525598));
#12315=CARTESIAN_POINT('Ctrl Pts',(11.7997807104374,1.34910745421534,-0.00105289019631603));
#12316=CARTESIAN_POINT('Ctrl Pts',(11.7891702365097,1.33854134055748,0.201406383632416));
#12317=CARTESIAN_POINT('Ctrl Pts',(11.7785598611315,1.32797539467558,0.403865671186622));
#12318=CARTESIAN_POINT('Ctrl Pts',(11.7679493857164,1.31740972279341,0.60632496775791));
#12319=CARTESIAN_POINT('Ctrl Pts',(11.7998379289556,1.32812520727701,-0.00214468456243374));
#12320=CARTESIAN_POINT('Ctrl Pts',(11.78922748064,1.31756145959839,0.200314730064766));
#12321=CARTESIAN_POINT('Ctrl Pts',(11.7786170316934,1.30699794333589,0.402774156733522));
#12322=CARTESIAN_POINT('Ctrl Pts',(11.7680065821063,1.2964346619681,0.605233595624295));
#12323=CARTESIAN_POINT('Ctrl Pts',(11.7680065821063,1.2964346619681,0.605233595624295));
#12324=CARTESIAN_POINT('Ctrl Pts',(11.7785795656372,1.30696064383315,0.403489051673192));
#12325=CARTESIAN_POINT('Ctrl Pts',(11.7891525485321,1.31748685893698,0.201744519857946));
#12326=CARTESIAN_POINT('Ctrl Pts',(11.7997255308004,1.32801330383774,3.10081821330854E-17));
#12327=CARTESIAN_POINT('Ctrl Pts',(11.3905090053564,1.32332268868375,0.7));
#12328=CARTESIAN_POINT('Ctrl Pts',(11.4830653488871,1.31448403714216,0.7));
#12329=CARTESIAN_POINT('Ctrl Pts',(11.5756099286391,1.3055179747114,0.7));
#12330=CARTESIAN_POINT('Ctrl Pts',(11.6681436286308,1.2964346619681,0.7));
#12331=CARTESIAN_POINT('Ctrl Pts',(11.3932507170007,1.35203326785047,0.7));
#12332=CARTESIAN_POINT('Ctrl Pts',(11.4858332859074,1.34318985044544,0.699999917777441));
#12333=CARTESIAN_POINT('Ctrl Pts',(11.5784027531871,1.33421922733773,0.700000082825348));
#12334=CARTESIAN_POINT('Ctrl Pts',(11.6709605510772,1.32513126902304,0.7));
#12335=CARTESIAN_POINT('Ctrl Pts',(11.3980029235658,1.40179729139028,0.67675176769038));
#12336=CARTESIAN_POINT('Ctrl Pts',(11.4906306781252,1.39294591144353,0.676755553516685));
#12337=CARTESIAN_POINT('Ctrl Pts',(11.583243842395,1.38396722707511,0.676759299309383));
#12338=CARTESIAN_POINT('Ctrl Pts',(11.6758431636759,1.37487151491717,0.676763114282959));
#12339=CARTESIAN_POINT('Ctrl Pts',(11.3998836071583,1.4214913811319,0.627256563056779));
#12340=CARTESIAN_POINT('Ctrl Pts',(11.4925297866457,1.41264104586547,0.627266369072496));
#12341=CARTESIAN_POINT('Ctrl Pts',(11.5851604051362,1.40366358810601,0.627276165220861));
#12342=CARTESIAN_POINT('Ctrl Pts',(11.6777767156198,1.39456903283364,0.627286048421068));
#12343=CARTESIAN_POINT('Ctrl Pts',(11.4,1.4227102204299,0.605660349289938));
#12344=CARTESIAN_POINT('Ctrl Pts',(11.4926474653491,1.41386220753305,0.605671932550561));
#12345=CARTESIAN_POINT('Ctrl Pts',(11.585279512325,1.40488700096013,0.605683574233495));
#12346=CARTESIAN_POINT('Ctrl Pts',(11.6778970386953,1.39579479040469,0.605695249702977));
#12347=CARTESIAN_POINT('Ctrl Pts',(0.200160078391861,1.15273809776858,-0.00218270663797729));
#12348=CARTESIAN_POINT('Ctrl Pts',(0.210771190526905,1.14220881798213,0.200289374419605));
#12349=CARTESIAN_POINT('Ctrl Pts',(0.221382303689445,1.13167991623912,0.402761475082968));
#12350=CARTESIAN_POINT('Ctrl Pts',(0.231993417893744,1.12115139781563,0.605233595624295));
#12351=CARTESIAN_POINT('Ctrl Pts',(0.200222527243758,1.17571472979894,-0.000991111558954063));
#12352=CARTESIAN_POINT('Ctrl Pts',(0.210833737189325,1.165180254798,0.201480665494204));
#12353=CARTESIAN_POINT('Ctrl Pts',(0.22144460713556,1.15464621893915,0.403952483115279));
#12354=CARTESIAN_POINT('Ctrl Pts',(0.232055819885544,1.1441124535127,0.606424296559433));
#12355=CARTESIAN_POINT('Ctrl Pts',(0.216855804290742,1.22156704800519,0.000521661548984882));
#12356=CARTESIAN_POINT('Ctrl Pts',(0.22745908713481,1.21102245544698,0.202993270772045));
#12357=CARTESIAN_POINT('Ctrl Pts',(0.238062502254218,1.2004779673848,0.405464877727456));
#12358=CARTESIAN_POINT('Ctrl Pts',(0.248665715176951,1.18993398276804,0.607936521147589));
#12359=CARTESIAN_POINT('Ctrl Pts',(0.258823218619159,1.24645290953083,-0.000383602721372307));
#12360=CARTESIAN_POINT('Ctrl Pts',(0.269410282911183,1.23591162135389,0.202088997034388));
#12361=CARTESIAN_POINT('Ctrl Pts',(0.279997195000074,1.22537100634993,0.404561639451295));
#12362=CARTESIAN_POINT('Ctrl Pts',(0.290584031570127,1.21483034200885,0.60703428203898));
#12363=CARTESIAN_POINT('Ctrl Pts',(0.281396145950812,1.25079993650842,-0.00134053860524368));
#12364=CARTESIAN_POINT('Ctrl Pts',(0.291976789318506,1.24026479669674,0.201132712115111));
#12365=CARTESIAN_POINT('Ctrl Pts',(0.302557285401186,1.22972999171968,0.403605987142707));
#12366=CARTESIAN_POINT('Ctrl Pts',(0.313137632044028,1.21919552599286,0.606079286803922));
#12367=CARTESIAN_POINT('Origin',(11.8002740930491,1.6,-0.0104671912485888));
#12368=CARTESIAN_POINT('Origin',(0.3318563713692,1.12115139781563,0.6));
#12369=CARTESIAN_POINT('',(0.331856371369203,1.12115139781563,0.9));
#12370=CARTESIAN_POINT('',(0.0322675109428288,1.12115139781563,0.615700786872883));
#12371=CARTESIAN_POINT('Origin',(0.3318563713692,1.12115139781563,0.6));
#12372=CARTESIAN_POINT('',(0.275700153393682,1.4152837823473,0.618237860411764));
#12373=CARTESIAN_POINT('Origin',(0.3318563713692,1.12115139781563,0.6));
#12374=CARTESIAN_POINT('Origin',(0.331856371369201,1.12115139781563,0.600000000000001));
#12375=CARTESIAN_POINT('Origin',(11.6681436286308,1.2964346619681,0.6));
#12376=CARTESIAN_POINT('',(11.6681436286308,1.2964346619681,0.9));
#12377=CARTESIAN_POINT('',(11.6974038588243,1.59451504727786,0.617085749108931));
#12378=CARTESIAN_POINT('Origin',(11.6681436286308,1.2964346619681,0.6));
#12379=CARTESIAN_POINT('',(11.9677324890572,1.2964346619681,0.615700786872884));
#12380=CARTESIAN_POINT('Origin',(11.6681436286308,1.2964346619681,0.6));
#12381=CARTESIAN_POINT('Origin',(11.6681436286308,1.2964346619681,0.6));
#12382=CARTESIAN_POINT('Origin',(0.3318563713692,-1.12115139781563,0.6));
#12383=CARTESIAN_POINT('',(0.3318563713692,-1.12115139781563,0.9));
#12384=CARTESIAN_POINT('',(0.27570015339368,-1.4152837823473,0.618237860411764));
#12385=CARTESIAN_POINT('Origin',(0.331856371369206,-1.12115139781563,0.6));
#12386=CARTESIAN_POINT('',(0.0322675109428289,-1.12115139781563,0.615700786872884));
#12387=CARTESIAN_POINT('Origin',(0.3318563713692,-1.12115139781563,0.6));
#12388=CARTESIAN_POINT('Origin',(0.331856371369201,-1.12115139781563,0.6));
#12389=CARTESIAN_POINT('Origin',(0.3318563713692,-0.7,0.6));
#12390=CARTESIAN_POINT('',(0.0322675109428288,-0.7,0.615700786872883));
#12391=CARTESIAN_POINT('',(0.3318563713692,-0.7,0.9));
#12392=CARTESIAN_POINT('Ctrl Pts',(0.243379792658812,-1.44768816351885,
-0.00386660544379547));
#12393=CARTESIAN_POINT('Ctrl Pts',(0.254153714020244,-1.43688644166428,
0.203501514337738));
#12394=CARTESIAN_POINT('Ctrl Pts',(0.264927169923045,-1.42608498030896,
0.410869669467268));
#12395=CARTESIAN_POINT('Ctrl Pts',(0.275700153393682,-1.4152837823473,0.618237860411764));
#12396=CARTESIAN_POINT('Ctrl Pts',(0.165985306518657,-1.43278556900406,
-0.000585522405354874));
#12397=CARTESIAN_POINT('Ctrl Pts',(0.176781886982148,-1.42196211044871,
0.206780297826791));
#12398=CARTESIAN_POINT('Ctrl Pts',(0.187577631459021,-1.41114055376332,
0.414146260476818));
#12399=CARTESIAN_POINT('Ctrl Pts',(0.198373523197449,-1.40031743725927,
0.621512129789107));
#12400=CARTESIAN_POINT('Ctrl Pts',(0.0420337764471552,-1.35067831466576,
0.00164062070145552));
#12401=CARTESIAN_POINT('Ctrl Pts',(0.0528811856485653,-1.33984924001505,
0.209003590924217));
#12402=CARTESIAN_POINT('Ctrl Pts',(0.0637288270387668,-1.3290196870647,
0.416366521726085));
#12403=CARTESIAN_POINT('Ctrl Pts',(0.0745760486629849,-1.31819094697801,
0.623729515932473));
#12404=CARTESIAN_POINT('Ctrl Pts',(-0.000174449685670057,-1.21258510413485,
-0.00332869829739982));
#12405=CARTESIAN_POINT('Ctrl Pts',(0.0106931634330696,-1.20178787588112,
0.204035045544629));
#12406=CARTESIAN_POINT('Ctrl Pts',(0.0215603573327632,-1.19099068058357,
0.411398812224037));
#12407=CARTESIAN_POINT('Ctrl Pts',(0.0324279732074593,-1.18019411246525,
0.618762589277523));
#12408=CARTESIAN_POINT('Ctrl Pts',(-0.000335035344191381,-1.15350137313465,
-0.00639285519773308));
#12409=CARTESIAN_POINT('Ctrl Pts',(0.0105324790023165,-1.1427176497384,
0.200971671503832));
#12410=CARTESIAN_POINT('Ctrl Pts',(0.0213999944262164,-1.13193432274319,
0.408336218763261));
#12411=CARTESIAN_POINT('Ctrl Pts',(0.0322675109428286,-1.12115139781563,
0.615700786872884));
#12412=CARTESIAN_POINT('Ctrl Pts',(0.243580684154575,-1.44748675362873,
-2.16840434497101E-17));
#12413=CARTESIAN_POINT('Ctrl Pts',(0.254287635915809,-1.43675217163244,
0.206079251738322));
#12414=CARTESIAN_POINT('Ctrl Pts',(0.264994127943615,-1.42601784692504,
0.412158538389471));
#12415=CARTESIAN_POINT('Ctrl Pts',(0.275700153393682,-1.4152837823473,0.618237860411764));
#12416=CARTESIAN_POINT('Ctrl Pts',(0.0322675109428286,-1.12115139781563,
0.615700786872884));
#12417=CARTESIAN_POINT('Ctrl Pts',(0.0215116728964671,-1.13182351356624,
0.410467170919192));
#12418=CARTESIAN_POINT('Ctrl Pts',(0.0107558359204751,-1.14249602316337,
0.205233575389367));
#12419=CARTESIAN_POINT('Ctrl Pts',(-1.41190227911925E-16,-1.15316892111333,
8.06646416329215E-17));
#12420=CARTESIAN_POINT('Origin',(11.6681436286308,-1.2964346619681,0.6));
#12421=CARTESIAN_POINT('',(11.9677324890572,-1.2964346619681,0.615700786872884));
#12422=CARTESIAN_POINT('',(11.6974038588243,-1.59451504727786,0.617085749108931));
#12423=CARTESIAN_POINT('Origin',(11.6681436286308,-1.2964346619681,0.600000000000001));
#12424=CARTESIAN_POINT('',(11.6681436286308,-1.2964346619681,0.9));
#12425=CARTESIAN_POINT('Origin',(11.6681436286308,-1.2964346619681,0.6));
#12426=CARTESIAN_POINT('Origin',(11.6681436286308,-1.2964346619681,0.6));
#12427=CARTESIAN_POINT('Origin',(11.6681436286308,0.8,0.6));
#12428=CARTESIAN_POINT('',(11.9677324890572,0.8,0.615700786872884));
#12429=CARTESIAN_POINT('',(11.6681436286308,0.8,0.9));
#12430=CARTESIAN_POINT('Ctrl Pts',(11.6681436286308,-1.2964346619681,0.9));
#12431=CARTESIAN_POINT('Ctrl Pts',(10.0505146497799,-1.45522470190849,0.9));
#12432=CARTESIAN_POINT('Ctrl Pts',(7.34698379851713,-1.66064017564263,0.9));
#12433=CARTESIAN_POINT('Ctrl Pts',(3.5507249968367,-1.5921338472202,0.9));
#12434=CARTESIAN_POINT('Ctrl Pts',(1.39628032950236,-1.32437289587156,0.9));
#12435=CARTESIAN_POINT('Ctrl Pts',(0.331856371369199,-1.12115139781563,
0.9));
#12436=CARTESIAN_POINT('Ctrl Pts',(11.6765943959699,-1.38252448313292,0.9));
#12437=CARTESIAN_POINT('Ctrl Pts',(10.0577014803155,-1.54155822929668,0.900004386952174));
#12438=CARTESIAN_POINT('Ctrl Pts',(7.35045927226653,-1.74750661992774,0.90000020513805));
#12439=CARTESIAN_POINT('Ctrl Pts',(3.54497585078588,-1.67885197560093,0.899998846478116));
#12440=CARTESIAN_POINT('Ctrl Pts',(1.38372480803625,-1.41002339692611,0.900007381454799));
#12441=CARTESIAN_POINT('Ctrl Pts',(0.315675209020016,-1.2059043252356,0.9));
#12442=CARTESIAN_POINT('Ctrl Pts',(11.6912432102654,-1.53175516862908,0.830242007927396));
#12443=CARTESIAN_POINT('Ctrl Pts',(10.070172518288,-1.69119563674726,0.830042231904815));
#12444=CARTESIAN_POINT('Ctrl Pts',(7.35645297288469,-1.89806162871739,0.829725685238203));
#12445=CARTESIAN_POINT('Ctrl Pts',(3.53503777381493,-1.8291593714544,0.829829026055289));
#12446=CARTESIAN_POINT('Ctrl Pts',(1.36192166831068,-1.55847530615989,0.830279056498203));
#12447=CARTESIAN_POINT('Ctrl Pts',(0.28762358730286,-1.35283178372728,0.830616544072481));
#12448=CARTESIAN_POINT('Ctrl Pts',(11.6970428895979,-1.59083777456472,0.681858145263203));
#12449=CARTESIAN_POINT('Ctrl Pts',(10.0750816081461,-1.75021732245097,0.681339641080976));
#12450=CARTESIAN_POINT('Ctrl Pts',(7.3588078744758,-1.95708146899443,0.680519979048775));
#12451=CARTESIAN_POINT('Ctrl Pts',(3.53113644431293,-1.88819699008302,0.68078748362792));
#12452=CARTESIAN_POINT('Ctrl Pts',(1.35331700817769,-1.61730376958615,0.681953432622034));
#12453=CARTESIAN_POINT('Ctrl Pts',(0.276437927844241,-1.41141950219787,
0.682830994206899));
#12454=CARTESIAN_POINT('Ctrl Pts',(11.6974038588243,-1.59451504727786,0.617085749108931));
#12455=CARTESIAN_POINT('Ctrl Pts',(10.0753786444688,-1.75377172884558,0.616473434532366));
#12456=CARTESIAN_POINT('Ctrl Pts',(7.35893161235257,-1.96044797105896,0.61550283428964));
#12457=CARTESIAN_POINT('Ctrl Pts',(3.53092277948893,-1.89162724517065,0.615818637525046));
#12458=CARTESIAN_POINT('Ctrl Pts',(1.35277799022997,-1.62098550016515,0.617200513836093));
#12459=CARTESIAN_POINT('Ctrl Pts',(0.27570015339368,-1.4152837823473,0.618237860411764));
#12460=CARTESIAN_POINT('Ctrl Pts',(0.27570015339368,-1.4152837823473,0.618237860411764));
#12461=CARTESIAN_POINT('Ctrl Pts',(1.35277799022997,-1.62098550016515,0.617200513836093));
#12462=CARTESIAN_POINT('Ctrl Pts',(3.53092277948893,-1.89162724517065,0.615818637525046));
#12463=CARTESIAN_POINT('Ctrl Pts',(7.35893161235257,-1.96044797105896,0.61550283428964));
#12464=CARTESIAN_POINT('Ctrl Pts',(10.0753786444688,-1.75377172884558,0.616473434532366));
#12465=CARTESIAN_POINT('Ctrl Pts',(11.6974038588243,-1.59451504727786,0.617085749108931));
#12466=CARTESIAN_POINT('Ctrl Pts',(11.6681436286308,-1.2964346619681,0.9));
#12467=CARTESIAN_POINT('Ctrl Pts',(10.0505146497799,-1.45522470190849,0.9));
#12468=CARTESIAN_POINT('Ctrl Pts',(7.34698379851713,-1.66064017564263,0.9));
#12469=CARTESIAN_POINT('Ctrl Pts',(3.5507249968367,-1.5921338472202,0.9));
#12470=CARTESIAN_POINT('Ctrl Pts',(1.39628032950236,-1.32437289587156,0.9));
#12471=CARTESIAN_POINT('Ctrl Pts',(0.331856371369199,-1.12115139781563,
0.9));
#12472=CARTESIAN_POINT('Ctrl Pts',(12.0003454972153,-1.32890342861544,-0.00659247958978532));
#12473=CARTESIAN_POINT('Ctrl Pts',(11.9894744951615,-1.31808026232082,0.200838596530835));
#12474=CARTESIAN_POINT('Ctrl Pts',(11.9786034924455,-1.30725733885828,0.408269685287046));
#12475=CARTESIAN_POINT('Ctrl Pts',(11.9677324890572,-1.2964346619681,0.615700786872884));
#12476=CARTESIAN_POINT('Ctrl Pts',(12.000116620981,-1.41283311850955,-0.00222526087931226));
#12477=CARTESIAN_POINT('Ctrl Pts',(11.9892453109784,-1.40200002127642,0.205205215027088));
#12478=CARTESIAN_POINT('Ctrl Pts',(11.9783750177566,-1.39116761830557,0.412635780645844));
#12479=CARTESIAN_POINT('Ctrl Pts',(11.9675037034976,-1.38033490526933,0.620066275407343));
#12480=CARTESIAN_POINT('Ctrl Pts',(11.9341774721098,-1.5584705948029,0.00191796595980313));
#12481=CARTESIAN_POINT('Ctrl Pts',(11.9233226835938,-1.54762133657986,0.209348350794306));
#12482=CARTESIAN_POINT('Ctrl Pts',(11.9124678718222,-1.53677206634062,0.416778732304926));
#12483=CARTESIAN_POINT('Ctrl Pts',(11.9016132473252,-1.52592301942363,0.624209134118803));
#12484=CARTESIAN_POINT('Ctrl Pts',(11.7925116537096,-1.62071287545028,-0.0022587989925734));
#12485=CARTESIAN_POINT('Ctrl Pts',(11.7816834491585,-1.6098745265243,0.205173499361722));
#12486=CARTESIAN_POINT('Ctrl Pts',(11.7708551999607,-1.59903658749835,0.41260581547062));
#12487=CARTESIAN_POINT('Ctrl Pts',(11.760027440985,-1.58819854843564,0.620038149897102));
#12488=CARTESIAN_POINT('Ctrl Pts',(11.7298629188572,-1.62699926142283,-0.0052140742384003));
#12489=CARTESIAN_POINT('Ctrl Pts',(11.7190429637906,-1.61617098622686,0.202219177289036));
#12490=CARTESIAN_POINT('Ctrl Pts',(11.708223275703,-1.60534291388117,0.409652451626141));
#12491=CARTESIAN_POINT('Ctrl Pts',(11.6974038588243,-1.59451504727786,0.617085749108931));
#12492=CARTESIAN_POINT('Ctrl Pts',(12.,-1.32855945177638,-1.94722710178397E-16));
#12493=CARTESIAN_POINT('Ctrl Pts',(11.9892441636707,-1.31785094954632,0.205233583190348));
#12494=CARTESIAN_POINT('Ctrl Pts',(11.978488326693,-1.30714268506935,0.410467178751997));
#12495=CARTESIAN_POINT('Ctrl Pts',(11.9677324890572,-1.2964346619681,0.615700786872884));
#12496=CARTESIAN_POINT('Ctrl Pts',(11.6974038588243,-1.59451504727786,0.617085749108931));
#12497=CARTESIAN_POINT('Ctrl Pts',(11.7081326228587,-1.605252190239,0.41139047675572));
#12498=CARTESIAN_POINT('Ctrl Pts',(11.7188616535763,-1.61598953550924,0.205695227161956));
#12499=CARTESIAN_POINT('Ctrl Pts',(11.7295909468525,-1.62672708026858,8.73866951023317E-17));
#12500=CARTESIAN_POINT('Ctrl Pts',(11.7298546566854,1.62699099289774,-0.00505567716946009));
#12501=CARTESIAN_POINT('Ctrl Pts',(11.719037455812,1.61616547398006,0.202324775346606));
#12502=CARTESIAN_POINT('Ctrl Pts',(11.7082205217827,1.60534015781013,0.409705250660816));
#12503=CARTESIAN_POINT('Ctrl Pts',(11.6974038588243,1.59451504727786,0.617085749108931));
#12504=CARTESIAN_POINT('Ctrl Pts',(11.8133862946664,1.61860913476435,-0.00111531114554236));
#12505=CARTESIAN_POINT('Ctrl Pts',(11.8025579038448,1.6077699189899,0.206263846261978));
#12506=CARTESIAN_POINT('Ctrl Pts',(11.7917299466398,1.59693199028804,0.41364309356145));
#12507=CARTESIAN_POINT('Ctrl Pts',(11.7809019683719,1.58609304882157,0.621022283493159));
#12508=CARTESIAN_POINT('Ctrl Pts',(11.9519653779615,1.53884931758497,0.00198566945999789));
#12509=CARTESIAN_POINT('Ctrl Pts',(11.9411087765487,1.52800449744246,0.209363119024413));
#12510=CARTESIAN_POINT('Ctrl Pts',(11.9302521502216,1.51715965702667,0.416740564833343));
#12511=CARTESIAN_POINT('Ctrl Pts',(11.9193956662674,1.50631506689811,0.624118030142866));
#12512=CARTESIAN_POINT('Ctrl Pts',(12.0001655389052,1.39184242582033,-0.00315867047762133));
#12513=CARTESIAN_POINT('Ctrl Pts',(11.9892972278067,1.38101476165208,0.204219175612729));
#12514=CARTESIAN_POINT('Ctrl Pts',(11.9784292129672,1.37018709651964,0.41159703650799));
#12515=CARTESIAN_POINT('Ctrl Pts',(11.9675608998875,1.35935984444403,0.618974903273729));
#12516=CARTESIAN_POINT('Ctrl Pts',(12.0003371960637,1.32889516399154,-0.00643408418199817));
#12517=CARTESIAN_POINT('Ctrl Pts',(11.9894689610601,1.31807475269516,0.200944193475792));
#12518=CARTESIAN_POINT('Ctrl Pts',(11.9786007253947,1.3072545841082,0.408322483762789));
#12519=CARTESIAN_POINT('Ctrl Pts',(11.9677324890572,1.2964346619681,0.615700786872884));
#12520=CARTESIAN_POINT('Ctrl Pts',(11.7295909468525,1.62672708026857,-8.50014503228635E-17));
#12521=CARTESIAN_POINT('Ctrl Pts',(11.7188616535763,1.61598953550924,0.205695227161956));
#12522=CARTESIAN_POINT('Ctrl Pts',(11.7081326228587,1.605252190239,0.411390476755719));
#12523=CARTESIAN_POINT('Ctrl Pts',(11.6974038588243,1.59451504727786,0.617085749108931));
#12524=CARTESIAN_POINT('Ctrl Pts',(11.9677324890572,1.2964346619681,0.615700786872884));
#12525=CARTESIAN_POINT('Ctrl Pts',(11.978488326693,1.30714268506935,0.410467178751997));
#12526=CARTESIAN_POINT('Ctrl Pts',(11.9892441636707,1.31785094954633,0.205233583190349));
#12527=CARTESIAN_POINT('Ctrl Pts',(12.,1.32855945177638,-2.38524477946811E-17));
#12528=CARTESIAN_POINT('Ctrl Pts',(0.3318563713692,1.12115139781563,0.9));
#12529=CARTESIAN_POINT('Ctrl Pts',(1.92849230856897,1.42598364489954,0.9));
#12530=CARTESIAN_POINT('Ctrl Pts',(5.71993880054687,1.76935652211139,0.9));
#12531=CARTESIAN_POINT('Ctrl Pts',(9.51130499016288,1.50815471522196,0.9));
#12532=CARTESIAN_POINT('Ctrl Pts',(11.6681436286308,1.2964346619681,0.9));
#12533=CARTESIAN_POINT('Ctrl Pts',(0.315675209020018,1.2059043252356,0.9));
#12534=CARTESIAN_POINT('Ctrl Pts',(1.91774960754439,1.51208293277137,0.900011072182198));
#12535=CARTESIAN_POINT('Ctrl Pts',(5.72069615836457,1.85663493780214,0.899990666655967));
#12536=CARTESIAN_POINT('Ctrl Pts',(9.5180705084307,1.59456947801794,0.900005849269565));
#12537=CARTESIAN_POINT('Ctrl Pts',(11.6765943959699,1.38252448313292,0.9));
#12538=CARTESIAN_POINT('Ctrl Pts',(0.287623587302861,1.35283178372728,0.83061654407248));
#12539=CARTESIAN_POINT('Ctrl Pts',(1.89907070881462,1.6612970673762,0.830110312711064));
#12540=CARTESIAN_POINT('Ctrl Pts',(5.72203120258494,2.00791989451774,0.829536565111056));
#12541=CARTESIAN_POINT('Ctrl Pts',(9.52981562096212,1.74434245945332,0.829975639897288));
#12542=CARTESIAN_POINT('Ctrl Pts',(11.6912432102654,1.53175516862908,0.830242007927395));
#12543=CARTESIAN_POINT('Ctrl Pts',(0.276437927844243,1.41141950219787,0.682830994206899));
#12544=CARTESIAN_POINT('Ctrl Pts',(1.89175654834445,1.7202459032803,0.681514651829601));
#12545=CARTESIAN_POINT('Ctrl Pts',(5.72254254462207,2.06699613896002,0.680031275065471));
#12546=CARTESIAN_POINT('Ctrl Pts',(9.53442784766217,1.80334383841306,0.681166806353567));
#12547=CARTESIAN_POINT('Ctrl Pts',(11.6970428895979,1.59083777456472,0.681858145263204));
#12548=CARTESIAN_POINT('Ctrl Pts',(0.275700153393682,1.4152837823473,0.618237860411764));
#12549=CARTESIAN_POINT('Ctrl Pts',(1.89131690864814,1.72383635907408,0.616681840548257));
#12550=CARTESIAN_POINT('Ctrl Pts',(5.72257555688819,2.07025489722917,0.614922376024419));
#12551=CARTESIAN_POINT('Ctrl Pts',(9.53470357301702,1.80685728936816,0.616269329673511));
#12552=CARTESIAN_POINT('Ctrl Pts',(11.6974038588243,1.59451504727786,0.617085749108931));
#12553=CARTESIAN_POINT('Ctrl Pts',(11.6974038588243,1.59451504727786,0.617085749108931));
#12554=CARTESIAN_POINT('Ctrl Pts',(9.53470357301702,1.80685728936816,0.616269329673511));
#12555=CARTESIAN_POINT('Ctrl Pts',(5.72257555688819,2.07025489722917,0.614922376024419));
#12556=CARTESIAN_POINT('Ctrl Pts',(1.89131690864814,1.72383635907408,0.616681840548257));
#12557=CARTESIAN_POINT('Ctrl Pts',(0.275700153393682,1.4152837823473,0.618237860411764));
#12558=CARTESIAN_POINT('Ctrl Pts',(0.3318563713692,1.12115139781563,0.9));
#12559=CARTESIAN_POINT('Ctrl Pts',(1.92849230856897,1.42598364489954,0.9));
#12560=CARTESIAN_POINT('Ctrl Pts',(5.71993880054687,1.76935652211139,0.9));
#12561=CARTESIAN_POINT('Ctrl Pts',(9.51130499016288,1.50815471522196,0.9));
#12562=CARTESIAN_POINT('Ctrl Pts',(11.6681436286308,1.2964346619681,0.9));
#12563=CARTESIAN_POINT('Ctrl Pts',(-0.000343174493958709,1.15350944952984,
-0.00654815942696785));
#12564=CARTESIAN_POINT('Ctrl Pts',(0.0105270529019337,1.14272303380391,
0.200868135340743));
#12565=CARTESIAN_POINT('Ctrl Pts',(0.0213972813757523,1.13193701467556,
0.408284450676511));
#12566=CARTESIAN_POINT('Ctrl Pts',(0.0322675109428289,1.12115139781563,
0.615700786872884));
#12567=CARTESIAN_POINT('Ctrl Pts',(-0.000129060241737355,1.23228777111366,
-0.0024626161135415));
#12568=CARTESIAN_POINT('Ctrl Pts',(0.0107416412387167,1.22148297235423,
0.204952596860618));
#12569=CARTESIAN_POINT('Ctrl Pts',(0.0216107531875107,1.21067920461451,
0.412367946918899));
#12570=CARTESIAN_POINT('Ctrl Pts',(0.0324814606290031,1.19987501734845,
0.61978319007907));
#12571=CARTESIAN_POINT('Ctrl Pts',(0.0574602827844584,1.36931747586956,
0.00164530659801973));
#12572=CARTESIAN_POINT('Ctrl Pts',(0.0683025556324749,1.35848226928888,
0.209060253413207));
#12573=CARTESIAN_POINT('Ctrl Pts',(0.079145272670006,1.34764679267913,0.416475160658282));
#12574=CARTESIAN_POINT('Ctrl Pts',(0.0899872847341513,1.33681188280878,
0.62389013300849));
#12575=CARTESIAN_POINT('Ctrl Pts',(0.185325846363896,1.43651931939441,-0.00156109881554352));
#12576=CARTESIAN_POINT('Ctrl Pts',(0.196119220517603,1.4256988926218,0.205857093047737));
#12577=CARTESIAN_POINT('Ctrl Pts',(0.20691256009293,1.41487906031557,0.413275315721495));
#12578=CARTESIAN_POINT('Ctrl Pts',(0.217705180746507,1.40405902353128,0.620693562444772));
#12579=CARTESIAN_POINT('Ctrl Pts',(0.243371723604776,1.44769625339383,-0.00402191236404));
#12580=CARTESIAN_POINT('Ctrl Pts',(0.254148334883323,1.43689183478419,0.203397976373256));
#12581=CARTESIAN_POINT('Ctrl Pts',(0.264924480472538,1.42608767680315,0.410817900476086));
#12582=CARTESIAN_POINT('Ctrl Pts',(0.275700153393682,1.4152837823473,0.618237860411764));
#12583=CARTESIAN_POINT('Ctrl Pts',(-1.23734572934908E-17,1.15316892111333,
-8.67361737988404E-19));
#12584=CARTESIAN_POINT('Ctrl Pts',(0.0107558359204753,1.14249602316336,
0.205233575389367));
#12585=CARTESIAN_POINT('Ctrl Pts',(0.0215116728964674,1.13182351356624,
0.410467170919192));
#12586=CARTESIAN_POINT('Ctrl Pts',(0.0322675109428289,1.12115139781563,
0.615700786872884));
#12587=CARTESIAN_POINT('Ctrl Pts',(0.275700153393682,1.4152837823473,0.618237860411764));
#12588=CARTESIAN_POINT('Ctrl Pts',(0.264994127943615,1.42601784692504,0.412158538389472));
#12589=CARTESIAN_POINT('Ctrl Pts',(0.254287635915814,1.43675217163244,0.206079251738322));
#12590=CARTESIAN_POINT('Ctrl Pts',(0.243580684154575,1.44748675362873,-1.9298798670242E-17));
#12591=CARTESIAN_POINT('Ctrl Pts',(11.7295909468525,-1.62672708026858,0.));
#12592=CARTESIAN_POINT('Ctrl Pts',(11.7192775324813,-1.61592692249094,0.206079286804135));
#12593=CARTESIAN_POINT('Ctrl Pts',(11.70896411811,-1.6051267647133,0.41215857360827));
#12594=CARTESIAN_POINT('Ctrl Pts',(11.6986507037388,-1.59432660693566,0.618237860412405));
#12595=CARTESIAN_POINT('Ctrl Pts',(7.90092085928651,-2.00057770191527,0.));
#12596=CARTESIAN_POINT('Ctrl Pts',(7.89749915175266,-1.98977754413763,0.206079286804135));
#12597=CARTESIAN_POINT('Ctrl Pts',(7.89407744421881,-1.97897738636,0.41215857360827));
#12598=CARTESIAN_POINT('Ctrl Pts',(7.89065573668496,-1.96817722858236,0.618237860412405));
#12599=CARTESIAN_POINT('Ctrl Pts',(4.07225077172054,-2.17467835246083,0.));
#12600=CARTESIAN_POINT('Ctrl Pts',(4.07572077102407,-2.16387819468319,0.206079286804135));
#12601=CARTESIAN_POINT('Ctrl Pts',(4.07919077032759,-2.15307803690555,0.41215857360827));
#12602=CARTESIAN_POINT('Ctrl Pts',(4.08266076963111,-2.14227787912792,0.618237860412405));
#12603=CARTESIAN_POINT('Ctrl Pts',(0.243580684154574,-1.44748675362873,
0.));
#12604=CARTESIAN_POINT('Ctrl Pts',(0.253942390295469,-1.43668659585109,
0.206079286804135));
#12605=CARTESIAN_POINT('Ctrl Pts',(0.264304096436365,-1.42588643807345,
0.41215857360827));
#12606=CARTESIAN_POINT('Ctrl Pts',(0.27466580257726,-1.41508628029581,0.618237860412405));
#12607=CARTESIAN_POINT('Origin',(0.,-1.4,0.));
#12608=CARTESIAN_POINT('Origin',(6.08012166120517,1.06803409199199E-16,
0.9));
#12609=CARTESIAN_POINT('Ctrl Pts',(0.243580684154574,1.44748675362873,0.));
#12610=CARTESIAN_POINT('Ctrl Pts',(0.253942390295469,1.43668659585109,0.206079286804135));
#12611=CARTESIAN_POINT('Ctrl Pts',(0.264304096436365,1.42588643807345,0.41215857360827));
#12612=CARTESIAN_POINT('Ctrl Pts',(0.27466580257726,1.41508628029581,0.618237860412405));
#12613=CARTESIAN_POINT('Ctrl Pts',(4.07225077172054,2.17467835246083,0.));
#12614=CARTESIAN_POINT('Ctrl Pts',(4.07572077102407,2.16387819468319,0.206079286804135));
#12615=CARTESIAN_POINT('Ctrl Pts',(4.07919077032759,2.15307803690555,0.41215857360827));
#12616=CARTESIAN_POINT('Ctrl Pts',(4.08266076963111,2.14227787912792,0.618237860412405));
#12617=CARTESIAN_POINT('Ctrl Pts',(7.90092085928651,2.00057770191527,0.));
#12618=CARTESIAN_POINT('Ctrl Pts',(7.89749915175266,1.98977754413763,0.206079286804135));
#12619=CARTESIAN_POINT('Ctrl Pts',(7.89407744421881,1.97897738636,0.41215857360827));
#12620=CARTESIAN_POINT('Ctrl Pts',(7.89065573668496,1.96817722858236,0.618237860412405));
#12621=CARTESIAN_POINT('Ctrl Pts',(11.7295909468525,1.62672708026858,0.));
#12622=CARTESIAN_POINT('Ctrl Pts',(11.7192775324813,1.61592692249094,0.206079286804135));
#12623=CARTESIAN_POINT('Ctrl Pts',(11.70896411811,1.6051267647133,0.41215857360827));
#12624=CARTESIAN_POINT('Ctrl Pts',(11.6986507037388,1.59432660693566,0.618237860412405));
#12625=CARTESIAN_POINT('Origin',(12.,1.6,0.));
#18336=UNCERTAINTY_MEASURE_WITH_UNIT(LENGTH_MEASURE(0.001),#18354,
'DISTANCE_ACCURACY_VALUE',
'Maximum model space distance between geometric entities at asserted c
onnectivities');
#18341=UNCERTAINTY_MEASURE_WITH_UNIT(LENGTH_MEASURE(0.001),#18354,
'DISTANCE_ACCURACY_VALUE',
'Maximum model space distance between geometric entities at asserted c
onnectivities');
#18348=(
GEOMETRIC_REPRESENTATION_CONTEXT(3)
GLOBAL_UNCERTAINTY_ASSIGNED_CONTEXT((#18336))
GLOBAL_UNIT_ASSIGNED_CONTEXT((#18354,#18356,#18357))
REPRESENTATION_CONTEXT('','3D')
);
#18353=(
GEOMETRIC_REPRESENTATION_CONTEXT(3)
GLOBAL_UNCERTAINTY_ASSIGNED_CONTEXT((#18341))
GLOBAL_UNIT_ASSIGNED_CONTEXT((#18354,#18356,#18357))
REPRESENTATION_CONTEXT('','3D')
);
#18354=(
LENGTH_UNIT()
NAMED_UNIT(*)
SI_UNIT(.CENTI.,.METRE.)
);
#18356=(
NAMED_UNIT(*)
PLANE_ANGLE_UNIT()
SI_UNIT($,.RADIAN.)
);
#18357=(
NAMED_UNIT(*)
SI_UNIT($,.STERADIAN.)
SOLID_ANGLE_UNIT()
);
#18364=SHAPE_DEFINITION_REPRESENTATION(#18375,#18402);
#18375=PRODUCT_DEFINITION_SHAPE('',$,#18414);
#18402=SHAPE_REPRESENTATION('',(#6788),#18348);
#18407=PRODUCT_DEFINITION_CONTEXT('part definition',#18442,'design');
#18414=PRODUCT_DEFINITION('2026-11-10-01-32-12-359',
'Lower structural shell',#18425,#18407);
#18425=PRODUCT_DEFINITION_FORMATION('',$,#18450);
#18442=APPLICATION_CONTEXT(
'Core Data for Automotive Mechanical Design Process');
#18443=PRODUCT_CONTEXT('part definition',#18442,'mechanical');
#18450=PRODUCT('2026-11-10-01-32-12-359','Lower structural shell',$,(#18443));
#18459=PRESENTATION_STYLE_ASSIGNMENT((#18467));
#18467=SURFACE_STYLE_USAGE(.BOTH.,#18475);
#18475=SURFACE_SIDE_STYLE('',(#18483));
#18483=SURFACE_STYLE_FILL_AREA(#18491);
#18491=FILL_AREA_STYLE('Structural dark blue',(#18499));
#18499=FILL_AREA_STYLE_COLOUR('Structural dark blue',#18507);
#18507=COLOUR_RGB('Structural dark blue',0.0901960784313725,0.270588235294118,
0.513725490196078);
ENDSEC;
END-ISO-10303-21;
